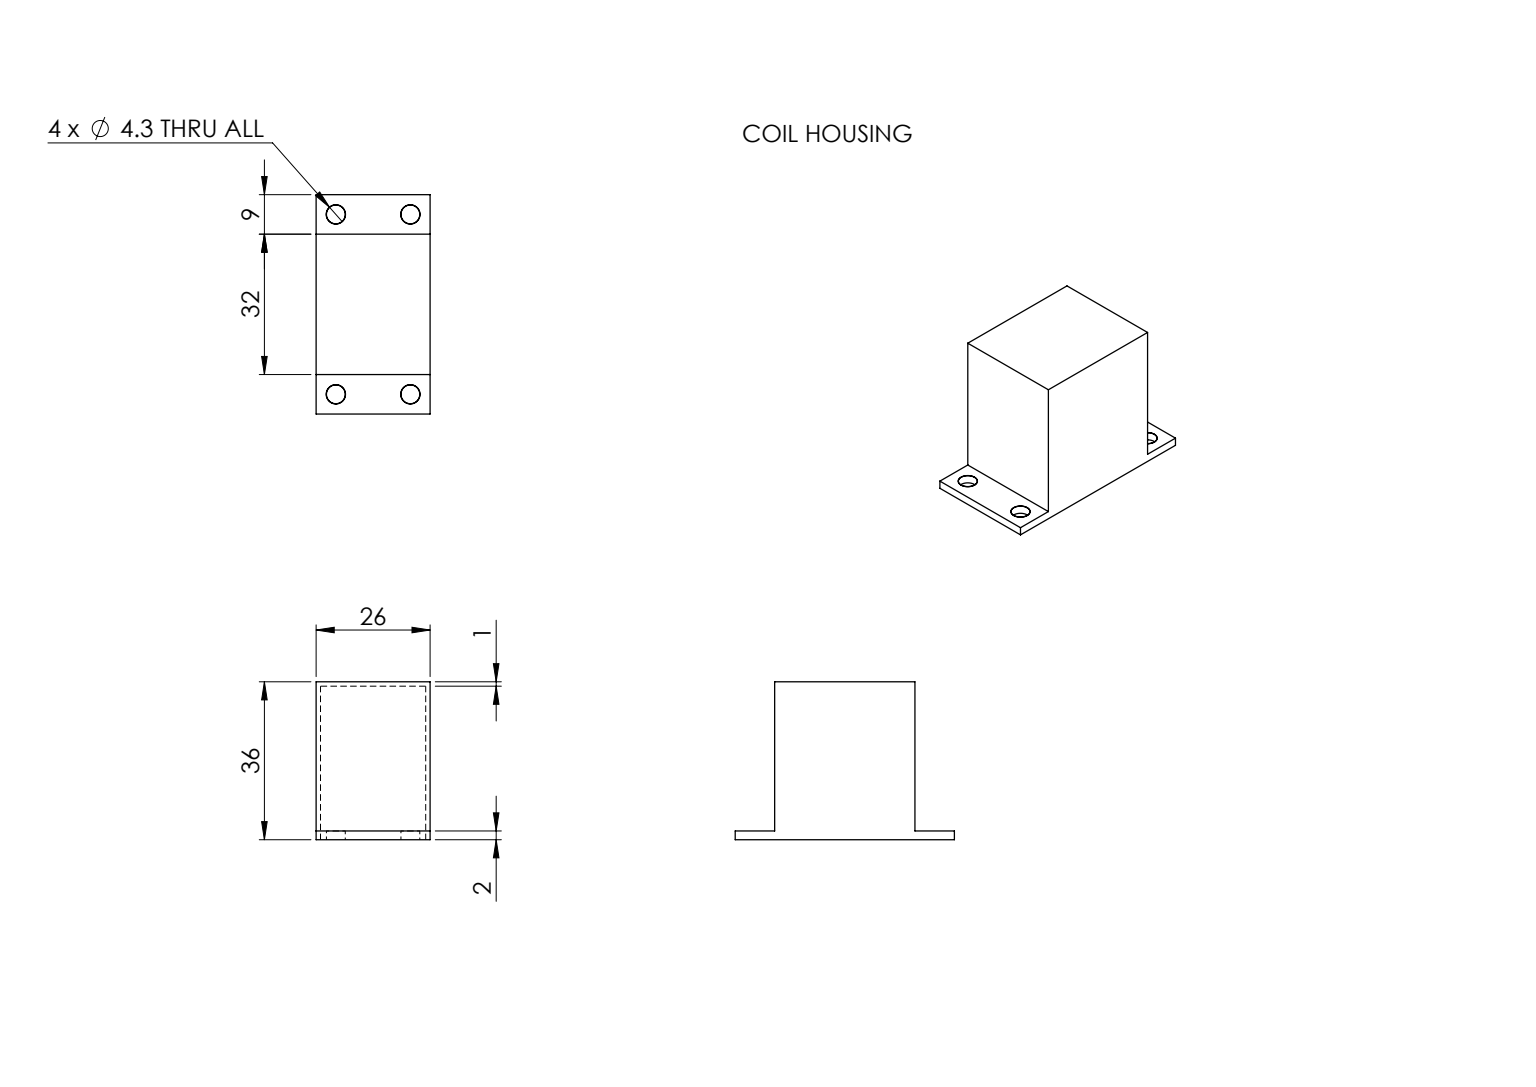
ISO-10303-21;
HEADER;
FILE_DESCRIPTION (('STEP AP214'),
    '1' );
FILE_NAME ('Coil Housing.step',
    '2026-10-25T16:39:07',
    ( '' ),
    ( '' ),
    'SwSTEP 2.0',
    'SolidWorks 2026',
    '' );
FILE_SCHEMA (( 'AUTOMOTIVE_DESIGN' ));
ENDSEC;

DATA;
#5=DIRECTION ( 'NONE',  ( -0.000000000000000000, 1.000000000000000000, -0.000000000000000000 ) ) ;
#11=LINE ( 'NONE', #8170, #4109 ) ;
#36=DIRECTION ( 'NONE',  ( 0.000000000000000000, 0.000000000000000000, 1.000000000000000000 ) ) ;
#41=CARTESIAN_POINT ( 'NONE',  ( -11.99999999999999822, 48.00000000000000000, 15.00000000000000000 ) ) ;
#55=ORIENTED_EDGE ( 'NONE', *, *, #17293, .T. ) ;
#160=VECTOR ( 'NONE', #10107, 1000.000000000000000 ) ;
#167=ORIENTED_EDGE ( 'NONE', *, *, #2613, .T. ) ;
#201=EDGE_CURVE ( 'NONE', #2949, #3217, #16754, .T. ) ;
#210=EDGE_CURVE ( 'NONE', #16170, #12849, #15356, .T. ) ;
#221=DIRECTION ( 'NONE',  ( -1.000000000000000000, 0.000000000000000000, 0.000000000000000000 ) ) ;
#243=CIRCLE ( 'NONE', #11190, 2.149999999999999023 ) ;
#258=DIRECTION ( 'NONE',  ( 0.000000000000000000, 0.000000000000000000, 1.000000000000000000 ) ) ;
#282=DIRECTION ( 'NONE',  ( 0.000000000000000000, 0.000000000000000000, -1.000000000000000000 ) ) ;
#297=VERTEX_POINT ( 'NONE', #12091 ) ;
#331=PLANE ( 'NONE',  #16743 ) ;
#386=FACE_OUTER_BOUND ( 'NONE', #16135, .T. ) ;
#409=ORIENTED_EDGE ( 'NONE', *, *, #7785, .F. ) ;
#452=DIRECTION ( 'NONE',  ( -0.000000000000000000, -0.000000000000000000, 1.000000000000000000 ) ) ;
#518=CARTESIAN_POINT ( 'NONE',  ( -8.500000000000007105, 14.80000000000000071, -20.49999999999999645 ) ) ;
#554=CARTESIAN_POINT ( 'NONE',  ( -8.500000000000007105, 15.00000000000000000, -20.49999999999999645 ) ) ;
#593=DIRECTION ( 'NONE',  ( 1.000000000000000000, 0.000000000000000000, 1.224646799147353207E-16 ) ) ;
#623=ORIENTED_EDGE ( 'NONE', *, *, #10806, .F. ) ;
#658=DIRECTION ( 'NONE',  ( 0.000000000000000000, 0.000000000000000000, 1.000000000000000000 ) ) ;
#706=DIRECTION ( 'NONE',  ( 0.000000000000000000, -0.000000000000000000, -1.000000000000000000 ) ) ;
#789=ADVANCED_FACE ( 'NONE', ( #9941 ), #12905, .F. ) ;
#800=ORIENTED_EDGE ( 'NONE', *, *, #7498, .F. ) ;
#842=EDGE_CURVE ( 'NONE', #9790, #6836, #12069, .T. ) ;
#872=ORIENTED_EDGE ( 'NONE', *, *, #16127, .F. ) ;
#958=DIRECTION ( 'NONE',  ( 0.000000000000000000, 0.000000000000000000, 1.000000000000000000 ) ) ;
#965=AXIS2_PLACEMENT_3D ( 'NONE', #17029, #8642, #1809 ) ;
#1016=TOROIDAL_SURFACE ( 'NONE', #15523, 2.200000000000000178, 0.2000000000000000111 ) ;
#1021=EDGE_LOOP ( 'NONE', ( #11107, #14324, #7812, #9618 ) ) ;
#1022=DIRECTION ( 'NONE',  ( -0.000000000000000000, 1.000000000000000000, -0.000000000000000000 ) ) ;
#1054=DIRECTION ( 'NONE',  ( -0.000000000000000000, 1.000000000000000000, -0.000000000000000000 ) ) ;
#1065=VECTOR ( 'NONE', #8366, 1000.000000000000000 ) ;
#1071=DIRECTION ( 'NONE',  ( -0.000000000000000000, 1.000000000000000000, -0.000000000000000000 ) ) ;
#1073=AXIS2_PLACEMENT_3D ( 'NONE', #1154, #15068, #6797 ) ;
#1078=CARTESIAN_POINT ( 'NONE',  ( 13.00000000000000178, 15.00000000000000178, -25.00000000000000355 ) ) ;
#1093=ORIENTED_EDGE ( 'NONE', *, *, #9929, .T. ) ;
#1099=FILL_AREA_STYLE ('',( #8400 ) ) ;
#1113=ADVANCED_FACE ( 'NONE', ( #1240 ), #4479, .T. ) ;
#1140=AXIS2_PLACEMENT_3D ( 'NONE', #6146, #11796, #10410 ) ;
#1154=CARTESIAN_POINT ( 'NONE',  ( -11.99999999999999822, 48.00000000000000000, -15.00000000000000000 ) ) ;
#1166=AXIS2_PLACEMENT_3D ( 'NONE', #8962, #12855, #8673 ) ;
#1183=DIRECTION ( 'NONE',  ( 0.000000000000000000, 0.000000000000000000, 1.000000000000000000 ) ) ;
#1194=SURFACE_STYLE_FILL_AREA ( #1099 ) ;
#1212=CARTESIAN_POINT ( 'NONE',  ( 8.500000000000001776, 13.00000000000000000, -22.64999999999999503 ) ) ;
#1216=FACE_OUTER_BOUND ( 'NONE', #16174, .T. ) ;
#1240=FACE_OUTER_BOUND ( 'NONE', #5632, .T. ) ;
#1252=ADVANCED_FACE ( 'NONE', ( #11227 ), #9922, .F. ) ;
#1254=DIRECTION ( 'NONE',  ( 1.000000000000000000, 0.000000000000000000, 0.000000000000000000 ) ) ;
#1264=CARTESIAN_POINT ( 'NONE',  ( -12.99999999999999822, 48.00000000000000000, -16.00000000000000000 ) ) ;
#1271=CARTESIAN_POINT ( 'NONE',  ( 8.500000000000001776, 14.99364916731036956, -20.49999999999999645 ) ) ;
#1277=EDGE_CURVE ( 'NONE', #11364, #9512, #18161, .T. ) ;
#1285=VERTEX_POINT ( 'NONE', #15594 ) ;
#1341=LINE ( 'NONE', #16656, #4429 ) ;
#1342=CYLINDRICAL_SURFACE ( 'NONE', #3202, 2.149999999999995470 ) ;
#1346=VERTEX_POINT ( 'NONE', #5580 ) ;
#1361=CARTESIAN_POINT ( 'NONE',  ( -8.500000000000010658, 14.99364916731036956, 18.34999999999999432 ) ) ;
#1362=AXIS2_PLACEMENT_3D ( 'NONE', #14070, #1651, #258 ) ;
#1388=ORIENTED_EDGE ( 'NONE', *, *, #14830, .T. ) ;
#1419=LINE ( 'NONE', #5668, #14928 ) ;
#1422=ORIENTED_EDGE ( 'NONE', *, *, #16477, .F. ) ;
#1456=CARTESIAN_POINT ( 'NONE',  ( -11.99999999999999822, 13.00000000000000178, -15.00000000000000000 ) ) ;
#1465=( LENGTH_UNIT ( ) NAMED_UNIT ( * ) SI_UNIT ( .MILLI., .METRE. ) );
#1466=DIRECTION ( 'NONE',  ( 1.000000000000000000, 0.000000000000000000, 0.000000000000000000 ) ) ;
#1468=ORIENTED_EDGE ( 'NONE', *, *, #10652, .T. ) ;
#1534=ORIENTED_EDGE ( 'NONE', *, *, #210, .T. ) ;
#1538=FACE_OUTER_BOUND ( 'NONE', #12873, .T. ) ;
#1551=FACE_OUTER_BOUND ( 'NONE', #4692, .T. ) ;
#1602=DIRECTION ( 'NONE',  ( -0.000000000000000000, 1.000000000000000000, -0.000000000000000000 ) ) ;
#1608=ADVANCED_FACE ( 'NONE', ( #1216 ), #3033, .T. ) ;
#1618=DIRECTION ( 'NONE',  ( 0.000000000000000000, 0.000000000000000000, 1.000000000000000000 ) ) ;
#1651=DIRECTION ( 'NONE',  ( -0.000000000000000000, 1.000000000000000000, -0.000000000000000000 ) ) ;
#1677=EDGE_CURVE ( 'NONE', #13721, #297, #14916, .T. ) ;
#1696=AXIS2_PLACEMENT_3D ( 'NONE', #10677, #16349, #958 ) ;
#1720=AXIS2_PLACEMENT_3D ( 'NONE', #7114, #5912, #15845 ) ;
#1733=VECTOR ( 'NONE', #3727, 1000.000000000000000 ) ;
#1761=VERTEX_POINT ( 'NONE', #17446 ) ;
#1765=VECTOR ( 'NONE', #16029, 1000.000000000000000 ) ;
#1789=DIRECTION ( 'NONE',  ( -0.000000000000000000, -1.000000000000000000, -0.000000000000000000 ) ) ;
#1809=DIRECTION ( 'NONE',  ( 0.000000000000000000, 0.000000000000000000, 1.000000000000000000 ) ) ;
#1819=DIRECTION ( 'NONE',  ( -0.000000000000000000, -1.000000000000000000, -0.000000000000000000 ) ) ;
#1884=EDGE_LOOP ( 'NONE', ( #14599, #5933, #16408, #14556 ) ) ;
#1885=STYLED_ITEM('',(#18389),#2427);
#1904=DIRECTION ( 'NONE',  ( -0.000000000000000000, -1.000000000000000000, -0.000000000000000000 ) ) ;
#1914=ORIENTED_EDGE ( 'NONE', *, *, #14897, .T. ) ;
#1942=FACE_OUTER_BOUND ( 'NONE', #17721, .T. ) ;
#1988=AXIS2_PLACEMENT_3D ( 'NONE', #15629, #5433, #11080 ) ;
#2022=DIRECTION ( 'NONE',  ( 0.000000000000000000, 0.000000000000000000, -1.000000000000000000 ) ) ;
#2058=DIRECTION ( 'NONE',  ( 1.000000000000000000, 0.000000000000000000, -0.000000000000000000 ) ) ;
#2063=CARTESIAN_POINT ( 'NONE',  ( 0.000000000000000000, 15.00000000000000178, 0.000000000000000000 ) ) ;
#2109=CARTESIAN_POINT ( 'NONE',  ( -12.99999999999999822, 48.00000000000000000, 16.00000000000000000 ) ) ;
#2150=ADVANCED_FACE ( 'NONE', ( #14013 ), #17441, .T. ) ;
#2189=CARTESIAN_POINT ( 'NONE',  ( -8.500000000000010658, 13.00000000000000000, 22.64999999999998437 ) ) ;
#2215=VERTEX_POINT ( 'NONE', #2810 ) ;
#2229=( LENGTH_UNIT ( ) NAMED_UNIT ( * ) SI_UNIT ( .MILLI., .METRE. ) );
#2242=EDGE_CURVE ( 'NONE', #6649, #8268, #1419, .T. ) ;
#2250=CARTESIAN_POINT ( 'NONE',  ( 8.499999999999992895, 14.80000000000000071, 20.49999999999999645 ) ) ;
#2266=DIRECTION ( 'NONE',  ( 0.000000000000000000, -1.000000000000000000, 0.000000000000000000 ) ) ;
#2310=CIRCLE ( 'NONE', #12648, 2.200000000000000622 ) ;
#2312=ADVANCED_FACE ( 'NONE', ( #7695 ), #13356, .F. ) ;
#2338=( LENGTH_UNIT ( ) NAMED_UNIT ( * ) SI_UNIT ( .MILLI., .METRE. ) );
#2378=CARTESIAN_POINT ( 'NONE',  ( 0.000000000000000000, 15.00000000000000178, 0.000000000000000000 ) ) ;
#2383=EDGE_CURVE ( 'NONE', #10239, #2662, #17878, .T. ) ;
#2403=VECTOR ( 'NONE', #17387, 1000.000000000000000 ) ;
#2408=( NAMED_UNIT ( * ) SI_UNIT ( $, .STERADIAN. ) SOLID_ANGLE_UNIT ( ) );
#2420=CARTESIAN_POINT ( 'NONE',  ( -8.500000000000010658, 13.00000000000000000, 20.49999999999998934 ) ) ;
#2421=DIRECTION ( 'NONE',  ( -0.000000000000000000, -1.000000000000000000, -0.000000000000000000 ) ) ;
#2425=FACE_OUTER_BOUND ( 'NONE', #4834, .T. ) ;
#2427=MANIFOLD_SOLID_BREP ( 'Cavity1', #15632 ) ;
#2469=CARTESIAN_POINT ( 'NONE',  ( -8.500000000000010658, 15.00000000000000178, 18.34999999999999432 ) ) ;
#2479=VECTOR ( 'NONE', #1789, 1000.000000000000000 ) ;
#2481=ORIENTED_EDGE ( 'NONE', *, *, #6992, .T. ) ;
#2500=DIRECTION ( 'NONE',  ( 0.000000000000000000, 0.000000000000000000, 1.000000000000000000 ) ) ;
#2503=LINE ( 'NONE', #16686, #9260 ) ;
#2535=CARTESIAN_POINT ( 'NONE',  ( 12.00000000000000178, 48.00000000000000000, 15.00000000000000000 ) ) ;
#2545=ORIENTED_EDGE ( 'NONE', *, *, #4076, .F. ) ;
#2552=DIRECTION ( 'NONE',  ( -0.000000000000000000, 1.000000000000000000, -0.000000000000000000 ) ) ;
#2553=CARTESIAN_POINT ( 'NONE',  ( 8.499999999999994671, 13.00000000000000000, 22.64999999999999503 ) ) ;
#2563=DIRECTION ( 'NONE',  ( 0.000000000000000000, -1.000000000000000000, 0.000000000000000000 ) ) ;
#2577=CARTESIAN_POINT ( 'NONE',  ( -8.500000000000010658, 14.80000000000000071, 20.49999999999998934 ) ) ;
#2597=ORIENTED_EDGE ( 'NONE', *, *, #842, .T. ) ;
#2598=CARTESIAN_POINT ( 'NONE',  ( -11.99999999999999822, 48.00000000000000000, 15.00000000000000000 ) ) ;
#2613=EDGE_CURVE ( 'NONE', #7280, #11197, #10033, .T. ) ;
#2652=EDGE_CURVE ( 'NONE', #13721, #9512, #7748, .T. ) ;
#2662=VERTEX_POINT ( 'NONE', #3290 ) ;
#2669=DIRECTION ( 'NONE',  ( 0.000000000000000000, 0.000000000000000000, 1.000000000000000000 ) ) ;
#2671=CARTESIAN_POINT ( 'NONE',  ( 8.499999999999994671, 14.99364916731036956, 22.64999999999999147 ) ) ;
#2679=SHAPE_REPRESENTATION_RELATIONSHIP ( 'NONE' , 'NONE' ,  #10877, #16698 ) ;
#2688=EDGE_CURVE ( 'NONE', #2662, #16507, #13972, .T. ) ;
#2698=CARTESIAN_POINT ( 'NONE',  ( 0.000000000000000000, 48.00000000000000000, 0.000000000000000000 ) ) ;
#2699=ORIENTED_EDGE ( 'NONE', *, *, #6147, .F. ) ;
#2721=CARTESIAN_POINT ( 'NONE',  ( -8.500000000000005329, 15.00000000000000178, -20.49999999999999645 ) ) ;
#2738=LINE ( 'NONE', #2469, #17193 ) ;
#2772=CARTESIAN_POINT ( 'NONE',  ( -13.00000000000000178, 15.00000000000000178, -25.00000000000000355 ) ) ;
#2775=ORIENTED_EDGE ( 'NONE', *, *, #17964, .T. ) ;
#2786=DIRECTION ( 'NONE',  ( 0.000000000000000000, -0.000000000000000000, -1.000000000000000000 ) ) ;
#2810=CARTESIAN_POINT ( 'NONE',  ( -13.00000000000000178, 15.00000000000000178, 25.00000000000000355 ) ) ;
#2812=DIRECTION ( 'NONE',  ( 0.000000000000000000, 0.000000000000000000, 1.000000000000000000 ) ) ;
#2844=VERTEX_POINT ( 'NONE', #7317 ) ;
#2889=DIRECTION ( 'NONE',  ( -0.000000000000000000, 1.000000000000000000, -0.000000000000000000 ) ) ;
#2909=CARTESIAN_POINT ( 'NONE',  ( 8.500000000000000000, 15.00000000000000000, -22.69999999999999929 ) ) ;
#2949=VERTEX_POINT ( 'NONE', #14676 ) ;
#2954=CARTESIAN_POINT ( 'NONE',  ( -11.99999999999999822, 48.00000000000000000, 15.00000000000000000 ) ) ;
#3012=CIRCLE ( 'NONE', #17864, 2.149999999999995470 ) ;
#3033=TOROIDAL_SURFACE ( 'NONE', #12497, 2.200000000000000178, 0.2000000000000000111 ) ;
#3038=ORIENTED_EDGE ( 'NONE', *, *, #16535, .T. ) ;
#3041=EDGE_CURVE ( 'NONE', #9856, #16492, #12322, .T. ) ;
#3042=ORIENTED_EDGE ( 'NONE', *, *, #1277, .T. ) ;
#3084=DIRECTION ( 'NONE',  ( 0.000000000000000000, 0.000000000000000000, 1.000000000000000000 ) ) ;
#3098=EDGE_LOOP ( 'NONE', ( #17464, #3426, #5820, #17938 ) ) ;
#3121=ORIENTED_EDGE ( 'NONE', *, *, #7037, .T. ) ;
#3170=ORIENTED_EDGE ( 'NONE', *, *, #10062, .T. ) ;
#3172=LINE ( 'NONE', #1264, #2479 ) ;
#3183=AXIS2_PLACEMENT_3D ( 'NONE', #2698, #11198, #2786 ) ;
#3184=DIRECTION ( 'NONE',  ( 0.000000000000000000, -1.000000000000000000, 0.000000000000000000 ) ) ;
#3185=VERTEX_POINT ( 'NONE', #10264 ) ;
#3190=FACE_OUTER_BOUND ( 'NONE', #10306, .T. ) ;
#3193=DIRECTION ( 'NONE',  ( 0.000000000000000000, -1.000000000000000000, 0.000000000000000000 ) ) ;
#3202=AXIS2_PLACEMENT_3D ( 'NONE', #8544, #15351, #17105 ) ;
#3209=DIRECTION ( 'NONE',  ( 0.000000000000000000, 0.000000000000000000, 1.000000000000000000 ) ) ;
#3217=VERTEX_POINT ( 'NONE', #6005 ) ;
#3239=ORIENTED_EDGE ( 'NONE', *, *, #2688, .F. ) ;
#3250=ORIENTED_EDGE ( 'NONE', *, *, #5910, .T. ) ;
#3290=CARTESIAN_POINT ( 'NONE',  ( 8.500000000000001776, 15.00000000000000000, -18.29999999999999716 ) ) ;
#3296=DIRECTION ( 'NONE',  ( 1.000000000000000000, 0.000000000000000000, -0.000000000000000000 ) ) ;
#3334=ORIENTED_EDGE ( 'NONE', *, *, #14608, .T. ) ;
#3340=ORIENTED_EDGE ( 'NONE', *, *, #12040, .T. ) ;
#3360=MECHANICAL_DESIGN_GEOMETRIC_PRESENTATION_REPRESENTATION('',(#1885),#7184);
#3381=ORIENTED_EDGE ( 'NONE', *, *, #14211, .F. ) ;
#3387=VECTOR ( 'NONE', #2552, 1000.000000000000000 ) ;
#3421=VERTEX_POINT ( 'NONE', #4810 ) ;
#3426=ORIENTED_EDGE ( 'NONE', *, *, #11240, .T. ) ;
#3440=EDGE_CURVE ( 'NONE', #5643, #9512, #12120, .T. ) ;
#3454=EDGE_CURVE ( 'NONE', #15329, #1285, #6590, .T. ) ;
#3534=DIRECTION ( 'NONE',  ( 0.000000000000000000, -0.000000000000000000, -1.000000000000000000 ) ) ;
#3598=ORIENTED_EDGE ( 'NONE', *, *, #4237, .T. ) ;
#3601=EDGE_CURVE ( 'NONE', #9347, #10311, #5169, .T. ) ;
#3625=DIRECTION ( 'NONE',  ( -0.000000000000000000, 1.000000000000000000, -0.000000000000000000 ) ) ;
#3635=AXIS2_PLACEMENT_3D ( 'NONE', #13994, #9900, #5554 ) ;
#3665=FACE_BOUND ( 'NONE', #3976, .T. ) ;
#3676=DIRECTION ( 'NONE',  ( 1.000000000000000000, 0.000000000000000000, 1.224646799147353207E-16 ) ) ;
#3682=CARTESIAN_POINT ( 'NONE',  ( -8.500000000000005329, 15.00000000000000178, -20.49999999999999645 ) ) ;
#3684=DIRECTION ( 'NONE',  ( 0.000000000000000000, 0.000000000000000000, -1.000000000000000000 ) ) ;
#3727=DIRECTION ( 'NONE',  ( -0.000000000000000000, 1.000000000000000000, -0.000000000000000000 ) ) ;
#3740=PLANE ( 'NONE',  #1073 ) ;
#3765=CYLINDRICAL_SURFACE ( 'NONE', #4714, 2.149999999999995470 ) ;
#3770=ORIENTED_EDGE ( 'NONE', *, *, #3041, .T. ) ;
#3778=( NAMED_UNIT ( * ) PLANE_ANGLE_UNIT ( ) SI_UNIT ( $, .RADIAN. ) );
#3790=LINE ( 'NONE', #15115, #18269 ) ;
#3818=ORIENTED_EDGE ( 'NONE', *, *, #12155, .T. ) ;
#3837=AXIS2_PLACEMENT_3D ( 'NONE', #11609, #8636, #36 ) ;
#3838=CARTESIAN_POINT ( 'NONE',  ( -13.00000000000000178, 49.00000000000000000, -16.00000000000000000 ) ) ;
#3883=VECTOR ( 'NONE', #15541, 1000.000000000000000 ) ;
#3904=ORIENTED_EDGE ( 'NONE', *, *, #7785, .T. ) ;
#3911=CYLINDRICAL_SURFACE ( 'NONE', #16250, 2.149999999999995470 ) ;
#3926=CARTESIAN_POINT ( 'NONE',  ( 8.500000000000001776, 14.99364916731036956, -22.64999999999999147 ) ) ;
#3933=FACE_OUTER_BOUND ( 'NONE', #1021, .T. ) ;
#3944=AXIS2_PLACEMENT_3D ( 'NONE', #17372, #10383, #9272 ) ;
#3976=EDGE_LOOP ( 'NONE', ( #17391, #409 ) ) ;
#3994=ORIENTED_EDGE ( 'NONE', *, *, #12650, .F. ) ;
#4010=DIRECTION ( 'NONE',  ( 0.000000000000000000, 0.000000000000000000, 1.000000000000000000 ) ) ;
#4022=CARTESIAN_POINT ( 'NONE',  ( -13.00000000000000178, 15.00000000000000178, -25.00000000000000355 ) ) ;
#4035=VECTOR ( 'NONE', #15160, 1000.000000000000000 ) ;
#4038=CARTESIAN_POINT ( 'NONE',  ( 8.499999999999992895, 14.80000000000000071, 22.69999999999999929 ) ) ;
#4062=VECTOR ( 'NONE', #16950, 1000.000000000000000 ) ;
#4065=PLANE ( 'NONE',  #3183 ) ;
#4069=( NAMED_UNIT ( * ) PLANE_ANGLE_UNIT ( ) SI_UNIT ( $, .RADIAN. ) );
#4071=ORIENTED_EDGE ( 'NONE', *, *, #6036, .F. ) ;
#4076=EDGE_CURVE ( 'NONE', #13129, #6514, #11073, .T. ) ;
#4104=LINE ( 'NONE', #12809, #1065 ) ;
#4109=VECTOR ( 'NONE', #6956, 1000.000000000000000 ) ;
#4135=CARTESIAN_POINT ( 'NONE',  ( 13.00000000000000178, 15.00000000000000178, 16.00000000000000000 ) ) ;
#4225=CARTESIAN_POINT ( 'NONE',  ( 13.00000000000000178, 49.00000000000000000, 16.00000000000000000 ) ) ;
#4237=EDGE_CURVE ( 'NONE', #4992, #6649, #3172, .T. ) ;
#4266=ORIENTED_EDGE ( 'NONE', *, *, #2242, .F. ) ;
#4267=DIRECTION ( 'NONE',  ( 0.000000000000000000, 0.000000000000000000, 1.000000000000000000 ) ) ;
#4280=DIRECTION ( 'NONE',  ( 0.000000000000000000, 0.000000000000000000, 1.000000000000000000 ) ) ;
#4286=LINE ( 'NONE', #9931, #160 ) ;
#4295=CARTESIAN_POINT ( 'NONE',  ( -13.00000000000000178, 49.00000000000000000, 16.00000000000000000 ) ) ;
#4319=SURFACE_STYLE_USAGE ( .BOTH. , #7095 ) ;
#4337=ORIENTED_EDGE ( 'NONE', *, *, #16762, .F. ) ;
#4365=AXIS2_PLACEMENT_3D ( 'NONE', #10794, #1071, #8008 ) ;
#4372=VECTOR ( 'NONE', #6715, 1000.000000000000000 ) ;
#4380=DIRECTION ( 'NONE',  ( -0.000000000000000000, -1.000000000000000000, -0.000000000000000000 ) ) ;
#4385=EDGE_LOOP ( 'NONE', ( #2545, #13867, #3250, #11309 ) ) ;
#4391=TOROIDAL_SURFACE ( 'NONE', #12673, 2.200000000000000178, 0.2000000000000000111 ) ;
#4429=VECTOR ( 'NONE', #12360, 1000.000000000000000 ) ;
#4479=TOROIDAL_SURFACE ( 'NONE', #17239, 2.200000000000000178, 0.2000000000000000111 ) ;
#4494=FACE_OUTER_BOUND ( 'NONE', #13704, .T. ) ;
#4520=LINE ( 'NONE', #11457, #17177 ) ;
#4565=LINE ( 'NONE', #12731, #2403 ) ;
#4633=CARTESIAN_POINT ( 'NONE',  ( -8.500000000000005329, 14.99364916731036956, -18.35000000000000142 ) ) ;
#4651=EDGE_CURVE ( 'NONE', #6401, #11263, #2503, .T. ) ;
#4684=VECTOR ( 'NONE', #282, 1000.000000000000000 ) ;
#4692=EDGE_LOOP ( 'NONE', ( #13063, #15901, #167, #9863 ) ) ;
#4710=VERTEX_POINT ( 'NONE', #2772 ) ;
#4714=AXIS2_PLACEMENT_3D ( 'NONE', #13224, #11834, #4795 ) ;
#4755=ORIENTED_EDGE ( 'NONE', *, *, #3440, .T. ) ;
#4758=APPLICATION_CONTEXT ( 'automotive_design' ) ;
#4759=ORIENTED_EDGE ( 'NONE', *, *, #2383, .F. ) ;
#4770=DIRECTION ( 'NONE',  ( -0.000000000000000000, 1.000000000000000000, -0.000000000000000000 ) ) ;
#4778=ORIENTED_EDGE ( 'NONE', *, *, #5020, .F. ) ;
#4795=DIRECTION ( 'NONE',  ( 0.000000000000000000, 0.000000000000000000, 1.000000000000000000 ) ) ;
#4801=ADVANCED_FACE ( 'NONE', ( #1551 ), #9965, .T. ) ;
#4807=DIRECTION ( 'NONE',  ( 0.000000000000000000, 0.000000000000000000, 1.000000000000000000 ) ) ;
#4810=CARTESIAN_POINT ( 'NONE',  ( -13.00000000000000178, 15.00000000000000178, 16.00000000000000000 ) ) ;
#4817=ORIENTED_EDGE ( 'NONE', *, *, #1277, .F. ) ;
#4823=DIRECTION ( 'NONE',  ( -0.000000000000000000, 1.000000000000000000, -0.000000000000000000 ) ) ;
#4831=CARTESIAN_POINT ( 'NONE',  ( 8.500000000000001776, 15.00000000000000000, -20.49999999999999645 ) ) ;
#4834=EDGE_LOOP ( 'NONE', ( #14359, #2699, #623, #14473 ) ) ;
#4845=AXIS2_PLACEMENT_3D ( 'NONE', #17879, #6540, #5148 ) ;
#4884=EDGE_CURVE ( 'NONE', #15656, #6744, #12847, .T. ) ;
#4891=ORIENTED_EDGE ( 'NONE', *, *, #11809, .T. ) ;
#4895=VERTEX_POINT ( 'NONE', #5803 ) ;
#4918=DIRECTION ( 'NONE',  ( -0.000000000000000000, 1.000000000000000000, -0.000000000000000000 ) ) ;
#4975=CARTESIAN_POINT ( 'NONE',  ( 8.500000000000001776, 15.00000000000000178, -20.49999999999999645 ) ) ;
#4992=VERTEX_POINT ( 'NONE', #12006 ) ;
#5020=EDGE_CURVE ( 'NONE', #10239, #6514, #12232, .T. ) ;
#5148=DIRECTION ( 'NONE',  ( 0.000000000000000000, 0.000000000000000000, 1.000000000000000000 ) ) ;
#5169=LINE ( 'NONE', #18175, #12206 ) ;
#5173=ORIENTED_EDGE ( 'NONE', *, *, #6036, .T. ) ;
#5221=LINE ( 'NONE', #9481, #3387 ) ;
#5240=ADVANCED_FACE ( 'NONE', ( #14995 ), #13769, .F. ) ;
#5260=CIRCLE ( 'NONE', #9695, 2.149999999999999023 ) ;
#5293=VERTEX_POINT ( 'NONE', #11158 ) ;
#5318=FACE_OUTER_BOUND ( 'NONE', #17771, .T. ) ;
#5319=CIRCLE ( 'NONE', #11217, 2.149999999999999023 ) ;
#5371=CARTESIAN_POINT ( 'NONE',  ( -11.99999999999999822, 48.00000000000000000, 15.00000000000000000 ) ) ;
#5387=VECTOR ( 'NONE', #15492, 1000.000000000000000 ) ;
#5433=DIRECTION ( 'NONE',  ( -0.000000000000000000, 1.000000000000000000, -0.000000000000000000 ) ) ;
#5487=ORIENTED_EDGE ( 'NONE', *, *, #9824, .F. ) ;
#5492=ORIENTED_EDGE ( 'NONE', *, *, #13638, .T. ) ;
#5526=EDGE_LOOP ( 'NONE', ( #13577, #4759 ) ) ;
#5551=ORIENTED_EDGE ( 'NONE', *, *, #210, .F. ) ;
#5554=DIRECTION ( 'NONE',  ( 0.000000000000000000, 0.000000000000000000, 1.000000000000000000 ) ) ;
#5562=VECTOR ( 'NONE', #4380, 1000.000000000000000 ) ;
#5580=CARTESIAN_POINT ( 'NONE',  ( 8.499999999999994671, 14.99364916731036956, 18.35000000000000142 ) ) ;
#5599=PRODUCT_DEFINITION ( 'UNKNOWN', '', #9538, #12661 ) ;
#5627=AXIS2_PLACEMENT_3D ( 'NONE', #8566, #13021, #13116 ) ;
#5632=EDGE_LOOP ( 'NONE', ( #5492, #13247, #12663, #3239 ) ) ;
#5643=VERTEX_POINT ( 'NONE', #2189 ) ;
#5668=CARTESIAN_POINT ( 'NONE',  ( -13.00000000000000178, 15.00000000000000178, -16.00000000000000000 ) ) ;
#5679=STYLED_ITEM ( 'NONE', ( #9793 ), #16698 ) ;
#5735=ORIENTED_EDGE ( 'NONE', *, *, #6017, .F. ) ;
#5756=LINE ( 'NONE', #17348, #8903 ) ;
#5759=ORIENTED_EDGE ( 'NONE', *, *, #2652, .T. ) ;
#5803=CARTESIAN_POINT ( 'NONE',  ( 8.499999999999994671, 13.00000000000000000, 18.34999999999999787 ) ) ;
#5820=ORIENTED_EDGE ( 'NONE', *, *, #7161, .F. ) ;
#5902=ADVANCED_FACE ( 'NONE', ( #5318 ), #1016, .T. ) ;
#5910=EDGE_CURVE ( 'NONE', #1761, #16507, #5221, .T. ) ;
#5912=DIRECTION ( 'NONE',  ( 1.000000000000000000, 0.000000000000000000, 1.224646799147353207E-16 ) ) ;
#5933=ORIENTED_EDGE ( 'NONE', *, *, #4076, .T. ) ;
#5936=DIRECTION ( 'NONE',  ( 0.000000000000000000, 0.000000000000000000, -1.000000000000000000 ) ) ;
#5968=CARTESIAN_POINT ( 'NONE',  ( 13.00000000000000178, 15.00000000000000178, -16.00000000000000000 ) ) ;
#5971=CARTESIAN_POINT ( 'NONE',  ( -11.99999999999999822, 48.00000000000000000, -15.00000000000000000 ) ) ;
#6005=CARTESIAN_POINT ( 'NONE',  ( 13.00000000000000178, 13.00000000000000178, -25.00000000000000355 ) ) ;
#6010=EDGE_CURVE ( 'NONE', #14506, #15334, #14986, .T. ) ;
#6017=EDGE_CURVE ( 'NONE', #6744, #3421, #4104, .T. ) ;
#6036=EDGE_CURVE ( 'NONE', #10707, #2844, #4286, .T. ) ;
#6085=VECTOR ( 'NONE', #14166, 1000.000000000000000 ) ;
#6097=ORIENTED_EDGE ( 'NONE', *, *, #14830, .F. ) ;
#6103=CIRCLE ( 'NONE', #16486, 2.200000000000000622 ) ;
#6107=EDGE_CURVE ( 'NONE', #3217, #9347, #15521, .T. ) ;
#6113=DIRECTION ( 'NONE',  ( 0.000000000000000000, -0.000000000000000000, 1.000000000000000000 ) ) ;
#6146=CARTESIAN_POINT ( 'NONE',  ( 0.000000000000000000, 13.00000000000000178, 0.000000000000000000 ) ) ;
#6147=EDGE_CURVE ( 'NONE', #10707, #9790, #7523, .T. ) ;
#6273=VERTEX_POINT ( 'NONE', #16821 ) ;
#6290=DIRECTION ( 'NONE',  ( 0.000000000000000000, 0.000000000000000000, 1.000000000000000000 ) ) ;
#6310=FACE_BOUND ( 'NONE', #8681, .T. ) ;
#6331=AXIS2_PLACEMENT_3D ( 'NONE', #10056, #1466, #7190 ) ;
#6340=ORIENTED_EDGE ( 'NONE', *, *, #12494, .F. ) ;
#6395=CARTESIAN_POINT ( 'NONE',  ( -11.99999999999999822, 48.00000000000000000, -15.00000000000000000 ) ) ;
#6401=VERTEX_POINT ( 'NONE', #2553 ) ;
#6418=CARTESIAN_POINT ( 'NONE',  ( -8.500000000000010658, 14.80000000000000071, 18.29999999999999005 ) ) ;
#6422=ORIENTED_EDGE ( 'NONE', *, *, #13298, .F. ) ;
#6428=DIRECTION ( 'NONE',  ( 1.000000000000000000, 0.000000000000000000, 0.000000000000000000 ) ) ;
#6473=ORIENTED_EDGE ( 'NONE', *, *, #10561, .F. ) ;
#6479=DIRECTION ( 'NONE',  ( 0.000000000000000000, -1.000000000000000000, 0.000000000000000000 ) ) ;
#6486=PRODUCT ( 'Coil Housing', 'Coil Housing', '', ( #17700 ) ) ;
#6488=AXIS2_PLACEMENT_3D ( 'NONE', #3682, #17886, #13324 ) ;
#6514=VERTEX_POINT ( 'NONE', #3926 ) ;
#6530=DIRECTION ( 'NONE',  ( 0.000000000000000000, 0.000000000000000000, 1.000000000000000000 ) ) ;
#6540=DIRECTION ( 'NONE',  ( -0.000000000000000000, 1.000000000000000000, -0.000000000000000000 ) ) ;
#6575=AXIS2_PLACEMENT_3D ( 'NONE', #11492, #9837, #12712 ) ;
#6589=ADVANCED_FACE ( 'NONE', ( #9757 ), #3740, .T. ) ;
#6590=CIRCLE ( 'NONE', #11603, 2.200000000000000622 ) ;
#6608=DIRECTION ( 'NONE',  ( 0.000000000000000000, 0.000000000000000000, 1.000000000000000000 ) ) ;
#6619=DIRECTION ( 'NONE',  ( -0.000000000000000000, 1.000000000000000000, -0.000000000000000000 ) ) ;
#6634=DIRECTION ( 'NONE',  ( -0.000000000000000000, 1.000000000000000000, -0.000000000000000000 ) ) ;
#6649=VERTEX_POINT ( 'NONE', #8447 ) ;
#6658=ORIENTED_EDGE ( 'NONE', *, *, #13615, .T. ) ;
#6708=DIRECTION ( 'NONE',  ( 0.000000000000000000, -1.000000000000000000, 0.000000000000000000 ) ) ;
#6715=DIRECTION ( 'NONE',  ( -0.000000000000000000, -1.000000000000000000, -0.000000000000000000 ) ) ;
#6744=VERTEX_POINT ( 'NONE', #17196 ) ;
#6752=DIRECTION ( 'NONE',  ( 0.000000000000000000, 0.000000000000000000, -1.000000000000000000 ) ) ;
#6776=DIRECTION ( 'NONE',  ( 1.000000000000000000, 0.000000000000000000, 0.000000000000000000 ) ) ;
#6797=DIRECTION ( 'NONE',  ( 1.000000000000000000, 0.000000000000000000, 0.000000000000000000 ) ) ;
#6820=DIRECTION ( 'NONE',  ( -0.000000000000000000, 1.000000000000000000, -0.000000000000000000 ) ) ;
#6836=VERTEX_POINT ( 'NONE', #9910 ) ;
#6849=ORIENTED_EDGE ( 'NONE', *, *, #9077, .T. ) ;
#6868=FACE_OUTER_BOUND ( 'NONE', #7471, .T. ) ;
#6933=ORIENTED_EDGE ( 'NONE', *, *, #13615, .F. ) ;
#6934=EDGE_CURVE ( 'NONE', #13129, #1761, #243, .T. ) ;
#6935=DIRECTION ( 'NONE',  ( 0.000000000000000000, 0.000000000000000000, 1.000000000000000000 ) ) ;
#6956=DIRECTION ( 'NONE',  ( 0.000000000000000000, 0.000000000000000000, -1.000000000000000000 ) ) ;
#6963=CARTESIAN_POINT ( 'NONE',  ( 8.499999999999992895, 14.80000000000000071, 20.49999999999999645 ) ) ;
#6972=DIRECTION ( 'NONE',  ( -0.000000000000000000, 1.000000000000000000, -0.000000000000000000 ) ) ;
#6990=FACE_OUTER_BOUND ( 'NONE', #13889, .T. ) ;
#6992=EDGE_CURVE ( 'NONE', #2844, #6836, #7219, .T. ) ;
#7013=AXIS2_PLACEMENT_3D ( 'NONE', #4038, #9688, #13962 ) ;
#7037=EDGE_CURVE ( 'NONE', #4895, #6401, #7060, .T. ) ;
#7060=CIRCLE ( 'NONE', #9726, 2.149999999999999023 ) ;
#7095=SURFACE_SIDE_STYLE ('',( #1194 ) ) ;
#7104=ORIENTED_EDGE ( 'NONE', *, *, #17293, .F. ) ;
#7110=PLANE ( 'NONE',  #17783 ) ;
#7114=CARTESIAN_POINT ( 'NONE',  ( -8.500000000000007105, 14.80000000000000071, -22.69999999999999929 ) ) ;
#7156=EDGE_CURVE ( 'NONE', #5293, #17312, #7686, .T. ) ;
#7161=EDGE_CURVE ( 'NONE', #11263, #1346, #10032, .T. ) ;
#7180=VECTOR ( 'NONE', #16055, 1000.000000000000000 ) ;
#7184=( GEOMETRIC_REPRESENTATION_CONTEXT ( 3 ) GLOBAL_UNCERTAINTY_ASSIGNED_CONTEXT ( ( #18263 ) ) GLOBAL_UNIT_ASSIGNED_CONTEXT ( ( #2338, #4069, #7874 ) ) REPRESENTATION_CONTEXT ( 'NONE', 'WORKASPACE' ) );
#7190=DIRECTION ( 'NONE',  ( 0.000000000000000000, 0.000000000000000000, -1.000000000000000000 ) ) ;
#7215=ORIENTED_EDGE ( 'NONE', *, *, #6010, .T. ) ;
#7219=LINE ( 'NONE', #11298, #4684 ) ;
#7280=VERTEX_POINT ( 'NONE', #6395 ) ;
#7317=CARTESIAN_POINT ( 'NONE',  ( 12.00000000000000178, 13.00000000000000178, 15.00000000000000000 ) ) ;
#7343=FACE_BOUND ( 'NONE', #16900, .T. ) ;
#7353=ORIENTED_EDGE ( 'NONE', *, *, #9800, .F. ) ;
#7381=CARTESIAN_POINT ( 'NONE',  ( -13.00000000000000178, 49.00000000000000000, 16.00000000000000000 ) ) ;
#7393=EDGE_LOOP ( 'NONE', ( #5735, #7617, #15124, #2775 ) ) ;
#7437=EDGE_CURVE ( 'NONE', #1761, #13129, #5319, .T. ) ;
#7458=DIRECTION ( 'NONE',  ( -0.000000000000000000, 1.000000000000000000, -0.000000000000000000 ) ) ;
#7471=EDGE_LOOP ( 'NONE', ( #3381, #16000, #10596, #6340 ) ) ;
#7474=ORIENTED_EDGE ( 'NONE', *, *, #8857, .T. ) ;
#7498=EDGE_CURVE ( 'NONE', #11197, #17312, #8323, .T. ) ;
#7502=PLANE ( 'NONE',  #11652 ) ;
#7509=FACE_BOUND ( 'NONE', #5526, .T. ) ;
#7523=LINE ( 'NONE', #16163, #17366 ) ;
#7535=PLANE ( 'NONE',  #1140 ) ;
#7549=CARTESIAN_POINT ( 'NONE',  ( 8.499999999999994671, 13.00000000000000000, 20.49999999999999645 ) ) ;
#7577=CARTESIAN_POINT ( 'NONE',  ( -8.500000000000010658, 15.00000000000000000, 22.69999999999999218 ) ) ;
#7617=ORIENTED_EDGE ( 'NONE', *, *, #4884, .F. ) ;
#7675=AXIS2_PLACEMENT_3D ( 'NONE', #12019, #3684, #11933 ) ;
#7678=VECTOR ( 'NONE', #8232, 1000.000000000000000 ) ;
#7686=LINE ( 'NONE', #10275, #16278 ) ;
#7688=LINE ( 'NONE', #17650, #7180 ) ;
#7695=FACE_OUTER_BOUND ( 'NONE', #13374, .T. ) ;
#7728=DIRECTION ( 'NONE',  ( 0.000000000000000000, 0.000000000000000000, 1.000000000000000000 ) ) ;
#7748=CIRCLE ( 'NONE', #17250, 0.1999999999999987899 ) ;
#7785=EDGE_CURVE ( 'NONE', #297, #13721, #8959, .T. ) ;
#7808=ORIENTED_EDGE ( 'NONE', *, *, #12676, .F. ) ;
#7812=ORIENTED_EDGE ( 'NONE', *, *, #12676, .T. ) ;
#7854=EDGE_LOOP ( 'NONE', ( #15580, #11538, #8532, #1093 ) ) ;
#7874=( NAMED_UNIT ( * ) SI_UNIT ( $, .STERADIAN. ) SOLID_ANGLE_UNIT ( ) );
#7875=DIRECTION ( 'NONE',  ( 0.000000000000000000, 0.000000000000000000, 1.000000000000000000 ) ) ;
#7917=LINE ( 'NONE', #2109, #11871 ) ;
#7956=EDGE_LOOP ( 'NONE', ( #14367, #4071, #8081, #2597 ) ) ;
#7990=CARTESIAN_POINT ( 'NONE',  ( 8.500000000000001776, 14.80000000000000071, -20.49999999999999645 ) ) ;
#8000=CARTESIAN_POINT ( 'NONE',  ( -8.500000000000007105, 14.80000000000000071, -20.49999999999999645 ) ) ;
#8008=DIRECTION ( 'NONE',  ( 0.000000000000000000, 0.000000000000000000, 1.000000000000000000 ) ) ;
#8052=AXIS2_PLACEMENT_3D ( 'NONE', #8616, #5936, #17090 ) ;
#8081=ORIENTED_EDGE ( 'NONE', *, *, #6147, .T. ) ;
#8122=CARTESIAN_POINT ( 'NONE',  ( -11.99999999999999822, 48.00000000000000000, 15.00000000000000000 ) ) ;
#8128=EDGE_LOOP ( 'NONE', ( #17895, #3121 ) ) ;
#8139=VERTEX_POINT ( 'NONE', #11345 ) ;
#8165=CIRCLE ( 'NONE', #1362, 2.200000000000000622 ) ;
#8168=EDGE_CURVE ( 'NONE', #4710, #6649, #9684, .T. ) ;
#8170=CARTESIAN_POINT ( 'NONE',  ( 13.00000000000000178, 13.00000000000000178, 0.000000000000000000 ) ) ;
#8190=EDGE_CURVE ( 'NONE', #6514, #16507, #3012, .T. ) ;
#8230=ORIENTED_EDGE ( 'NONE', *, *, #12650, .T. ) ;
#8232=DIRECTION ( 'NONE',  ( -0.000000000000000000, -1.000000000000000000, -0.000000000000000000 ) ) ;
#8233=ADVANCED_FACE ( 'NONE', ( #1538 ), #331, .F. ) ;
#8268=VERTEX_POINT ( 'NONE', #5968 ) ;
#8295=EDGE_CURVE ( 'NONE', #8139, #8268, #14418, .T. ) ;
#8323=LINE ( 'NONE', #2598, #7678 ) ;
#8329=CARTESIAN_POINT ( 'NONE',  ( 8.499999999999992895, 15.00000000000000000, 20.49999999999999645 ) ) ;
#8335=COLOUR_RGB ( '',0.8941176470588234615, 0.8941176470588234615, 0.8941176470588234615 ) ;
#8366=DIRECTION ( 'NONE',  ( -1.000000000000000000, -0.000000000000000000, -0.000000000000000000 ) ) ;
#8386=CARTESIAN_POINT ( 'NONE',  ( 8.499999999999992895, 15.00000000000000000, 20.49999999999999645 ) ) ;
#8400=FILL_AREA_STYLE_COLOUR ( '', #8335 ) ;
#8435=DIRECTION ( 'NONE',  ( -0.000000000000000000, 1.000000000000000000, -0.000000000000000000 ) ) ;
#8447=CARTESIAN_POINT ( 'NONE',  ( -12.99999999999999822, 15.00000000000000000, -16.00000000000000000 ) ) ;
#8492=LINE ( 'NONE', #7381, #6085 ) ;
#8532=ORIENTED_EDGE ( 'NONE', *, *, #16511, .T. ) ;
#8544=CARTESIAN_POINT ( 'NONE',  ( -8.500000000000010658, 15.00000000000000178, 20.49999999999998934 ) ) ;
#8554=CARTESIAN_POINT ( 'NONE',  ( -13.00000000000000178, 13.00000000000000178, -25.00000000000000355 ) ) ;
#8562=DIRECTION ( 'NONE',  ( 0.000000000000000000, 0.000000000000000000, -1.000000000000000000 ) ) ;
#8565=ADVANCED_FACE ( 'NONE', ( #13524 ), #7502, .F. ) ;
#8566=CARTESIAN_POINT ( 'NONE',  ( 8.499999999999992895, 14.99364916731036956, 20.49999999999999645 ) ) ;
#8616=CARTESIAN_POINT ( 'NONE',  ( -13.00000000000000178, 15.00000000000000178, 25.00000000000000355 ) ) ;
#8620=EDGE_CURVE ( 'NONE', #17312, #2844, #7688, .T. ) ;
#8636=DIRECTION ( 'NONE',  ( -0.000000000000000000, 1.000000000000000000, -0.000000000000000000 ) ) ;
#8642=DIRECTION ( 'NONE',  ( -1.000000000000000000, 0.000000000000000000, 0.000000000000000000 ) ) ;
#8649=AXIS2_PLACEMENT_3D ( 'NONE', #11131, #9741, #15422 ) ;
#8651=CARTESIAN_POINT ( 'NONE',  ( -13.00000000000000178, 15.00000000000000178, -16.00000000000000000 ) ) ;
#8654=LINE ( 'NONE', #11261, #4062 ) ;
#8667=ORIENTED_EDGE ( 'NONE', *, *, #2688, .T. ) ;
#8673=DIRECTION ( 'NONE',  ( 0.000000000000000000, 0.000000000000000000, -1.000000000000000000 ) ) ;
#8681=EDGE_LOOP ( 'NONE', ( #9439, #10411 ) ) ;
#8742=EDGE_CURVE ( 'NONE', #12849, #16170, #17278, .T. ) ;
#8762=ORIENTED_EDGE ( 'NONE', *, *, #3041, .F. ) ;
#8807=AXIS2_PLACEMENT_3D ( 'NONE', #8329, #13904, #6935 ) ;
#8829=FACE_BOUND ( 'NONE', #9067, .T. ) ;
#8857=EDGE_CURVE ( 'NONE', #2215, #10311, #3790, .T. ) ;
#8903=VECTOR ( 'NONE', #452, 1000.000000000000000 ) ;
#8959=CIRCLE ( 'NONE', #10123, 2.200000000000000622 ) ;
#8962=CARTESIAN_POINT ( 'NONE',  ( 8.499999999999992895, 14.80000000000000071, 18.29999999999999716 ) ) ;
#8967=EDGE_CURVE ( 'NONE', #1285, #15329, #8165, .T. ) ;
#8969=AXIS2_PLACEMENT_3D ( 'NONE', #4831, #4918, #13166 ) ;
#8986=AXIS2_PLACEMENT_3D ( 'NONE', #10340, #3676, #2022 ) ;
#8999=EDGE_LOOP ( 'NONE', ( #11746, #800, #12211, #5173 ) ) ;
#9020=CARTESIAN_POINT ( 'NONE',  ( 12.00000000000000178, 48.00000000000000000, -15.00000000000000000 ) ) ;
#9024=CARTESIAN_POINT ( 'NONE',  ( 0.000000000000000000, 0.000000000000000000, 0.000000000000000000 ) ) ;
#9050=ORIENTED_EDGE ( 'NONE', *, *, #13460, .T. ) ;
#9065=CARTESIAN_POINT ( 'NONE',  ( 8.500000000000001776, 15.00000000000000000, -20.49999999999999645 ) ) ;
#9067=EDGE_LOOP ( 'NONE', ( #2481, #15038, #13597, #9733 ) ) ;
#9077=EDGE_CURVE ( 'NONE', #13832, #15656, #8492, .T. ) ;
#9141=APPLICATION_CONTEXT ( 'automotive_design' ) ;
#9146=ADVANCED_FACE ( 'NONE', ( #15932 ), #17711, .F. ) ;
#9147=CIRCLE ( 'NONE', #1166, 0.1999999999999987899 ) ;
#9260=VECTOR ( 'NONE', #12214, 1000.000000000000000 ) ;
#9270=ORIENTED_EDGE ( 'NONE', *, *, #10062, .F. ) ;
#9272=DIRECTION ( 'NONE',  ( 0.000000000000000000, 0.000000000000000000, -1.000000000000000000 ) ) ;
#9291=ORIENTED_EDGE ( 'NONE', *, *, #15618, .F. ) ;
#9347=VERTEX_POINT ( 'NONE', #8554 ) ;
#9372=AXIS2_PLACEMENT_3D ( 'NONE', #2577, #15277, #2669 ) ;
#9380=CARTESIAN_POINT ( 'NONE',  ( -8.500000000000005329, 13.00000000000000000, -18.35000000000000142 ) ) ;
#9439=ORIENTED_EDGE ( 'NONE', *, *, #8967, .F. ) ;
#9476=CIRCLE ( 'NONE', #5627, 2.149999999999995470 ) ;
#9481=CARTESIAN_POINT ( 'NONE',  ( 8.500000000000001776, 15.00000000000000178, -18.35000000000000142 ) ) ;
#9512=VERTEX_POINT ( 'NONE', #14827 ) ;
#9528=UNCERTAINTY_MEASURE_WITH_UNIT (LENGTH_MEASURE( 1.000000000000000082E-05 ), #1465, 'distance_accuracy_value', 'NONE');
#9532=DIRECTION ( 'NONE',  ( 0.000000000000000000, 0.000000000000000000, 1.000000000000000000 ) ) ;
#9538=PRODUCT_DEFINITION_FORMATION_WITH_SPECIFIED_SOURCE ( 'ANY', '', #6486, .NOT_KNOWN. ) ;
#9587=DIRECTION ( 'NONE',  ( -0.000000000000000000, 1.000000000000000000, -0.000000000000000000 ) ) ;
#9618=ORIENTED_EDGE ( 'NONE', *, *, #9800, .T. ) ;
#9657=ADVANCED_FACE ( 'NONE', ( #12564 ), #10840, .T. ) ;
#9663=AXIS2_PLACEMENT_3D ( 'NONE', #518, #4770, #10423 ) ;
#9670=CIRCLE ( 'NONE', #1696, 0.1999999999999987899 ) ;
#9684=LINE ( 'NONE', #8651, #3883 ) ;
#9686=LINE ( 'NONE', #4135, #13515 ) ;
#9688=DIRECTION ( 'NONE',  ( -1.000000000000000000, 0.000000000000000000, 0.000000000000000000 ) ) ;
#9695=AXIS2_PLACEMENT_3D ( 'NONE', #7549, #16104, #13203 ) ;
#9709=AXIS2_PLACEMENT_3D ( 'NONE', #17301, #3184, #11790 ) ;
#9723=AXIS2_PLACEMENT_3D ( 'NONE', #2420, #4823, #10471 ) ;
#9726=AXIS2_PLACEMENT_3D ( 'NONE', #10182, #15859, #4267 ) ;
#9727=EDGE_CURVE ( 'NONE', #17654, #6273, #6103, .T. ) ;
#9733=ORIENTED_EDGE ( 'NONE', *, *, #8620, .T. ) ;
#9741=DIRECTION ( 'NONE',  ( -1.000000000000000000, 0.000000000000000000, 0.000000000000000000 ) ) ;
#9757=FACE_OUTER_BOUND ( 'NONE', #7854, .T. ) ;
#9769=ADVANCED_FACE ( 'NONE', ( #6990 ), #16947, .F. ) ;
#9790=VERTEX_POINT ( 'NONE', #16766 ) ;
#9793=PRESENTATION_STYLE_ASSIGNMENT (( #4319 ) ) ;
#9800=EDGE_CURVE ( 'NONE', #9856, #6744, #9686, .T. ) ;
#9805=DIRECTION ( 'NONE',  ( -1.000000000000000000, 0.000000000000000000, -0.000000000000000000 ) ) ;
#9824=EDGE_CURVE ( 'NONE', #15656, #8139, #11259, .T. ) ;
#9825=( GEOMETRIC_REPRESENTATION_CONTEXT ( 3 ) GLOBAL_UNCERTAINTY_ASSIGNED_CONTEXT ( ( #9528 ) ) GLOBAL_UNIT_ASSIGNED_CONTEXT ( ( #1465, #13973, #12574 ) ) REPRESENTATION_CONTEXT ( 'NONE', 'WORKASPACE' ) );
#9837=DIRECTION ( 'NONE',  ( 0.000000000000000000, -1.000000000000000000, 0.000000000000000000 ) ) ;
#9856=VERTEX_POINT ( 'NONE', #10043 ) ;
#9863=ORIENTED_EDGE ( 'NONE', *, *, #7498, .T. ) ;
#9868=DIRECTION ( 'NONE',  ( 0.000000000000000000, 0.000000000000000000, -1.000000000000000000 ) ) ;
#9892=FACE_OUTER_BOUND ( 'NONE', #8999, .T. ) ;
#9900=DIRECTION ( 'NONE',  ( -0.000000000000000000, 1.000000000000000000, -0.000000000000000000 ) ) ;
#9910=CARTESIAN_POINT ( 'NONE',  ( 12.00000000000000178, 13.00000000000000178, -15.00000000000000000 ) ) ;
#9916=LINE ( 'NONE', #15423, #13565 ) ;
#9922=PLANE ( 'NONE',  #8052 ) ;
#9929=EDGE_CURVE ( 'NONE', #7280, #5293, #13020, .T. ) ;
#9931=CARTESIAN_POINT ( 'NONE',  ( 12.00000000000000178, 48.00000000000000000, 15.00000000000000000 ) ) ;
#9937=CARTESIAN_POINT ( 'NONE',  ( -13.00000000000000178, 13.00000000000000178, 25.00000000000000355 ) ) ;
#9941=FACE_OUTER_BOUND ( 'NONE', #3098, .T. ) ;
#9942=ORIENTED_EDGE ( 'NONE', *, *, #8857, .F. ) ;
#9965=PLANE ( 'NONE',  #6331 ) ;
#9981=ORIENTED_EDGE ( 'NONE', *, *, #13298, .T. ) ;
#9985=EDGE_LOOP ( 'NONE', ( #8230, #17134, #6097, #11274, #5487, #11548, #7353, #3770 ) ) ;
#9988=ADVANCED_FACE ( 'NONE', ( #4494 ), #16189, .T. ) ;
#10032=CIRCLE ( 'NONE', #12995, 2.149999999999995470 ) ;
#10033=LINE ( 'NONE', #41, #15749 ) ;
#10043=CARTESIAN_POINT ( 'NONE',  ( 13.00000000000000178, 15.00000000000000178, 25.00000000000000355 ) ) ;
#10046=LINE ( 'NONE', #1456, #13541 ) ;
#10056=CARTESIAN_POINT ( 'NONE',  ( -11.99999999999999822, 48.00000000000000000, 15.00000000000000000 ) ) ;
#10062=EDGE_CURVE ( 'NONE', #8139, #4992, #17602, .T. ) ;
#10107=DIRECTION ( 'NONE',  ( -0.000000000000000000, -1.000000000000000000, -0.000000000000000000 ) ) ;
#10123=AXIS2_PLACEMENT_3D ( 'NONE', #17430, #10534, #13223 ) ;
#10134=CARTESIAN_POINT ( 'NONE',  ( -13.00000000000000178, 15.00000000000000178, -25.00000000000000355 ) ) ;
#10182=CARTESIAN_POINT ( 'NONE',  ( 8.499999999999994671, 13.00000000000000000, 20.49999999999999645 ) ) ;
#10219=VECTOR ( 'NONE', #11321, 1000.000000000000000 ) ;
#10239=VERTEX_POINT ( 'NONE', #2909 ) ;
#10244=CARTESIAN_POINT ( 'NONE',  ( 13.00000000000000178, 48.00000000000000000, 16.00000000000000000 ) ) ;
#10264=CARTESIAN_POINT ( 'NONE',  ( -8.500000000000010658, 13.00000000000000000, 18.34999999999999432 ) ) ;
#10275=CARTESIAN_POINT ( 'NONE',  ( -11.99999999999999822, 13.00000000000000178, 15.00000000000000000 ) ) ;
#10306=EDGE_LOOP ( 'NONE', ( #3994, #1422, #13152, #15596 ) ) ;
#10311=VERTEX_POINT ( 'NONE', #9937 ) ;
#10340=CARTESIAN_POINT ( 'NONE',  ( 8.500000000000001776, 14.80000000000000071, -22.69999999999999929 ) ) ;
#10374=CARTESIAN_POINT ( 'NONE',  ( 8.499999999999992895, 14.99364916731036956, 20.49999999999999645 ) ) ;
#10383=DIRECTION ( 'NONE',  ( 1.000000000000000000, 0.000000000000000000, 0.000000000000000000 ) ) ;
#10404=DIRECTION ( 'NONE',  ( 0.000000000000000000, -0.000000000000000000, -1.000000000000000000 ) ) ;
#10410=DIRECTION ( 'NONE',  ( 0.000000000000000000, -0.000000000000000000, 1.000000000000000000 ) ) ;
#10411=ORIENTED_EDGE ( 'NONE', *, *, #3454, .F. ) ;
#10423=DIRECTION ( 'NONE',  ( 0.000000000000000000, 0.000000000000000000, 1.000000000000000000 ) ) ;
#10443=EDGE_LOOP ( 'NONE', ( #16379, #6422 ) ) ;
#10471=DIRECTION ( 'NONE',  ( 0.000000000000000000, 0.000000000000000000, 1.000000000000000000 ) ) ;
#10495=FACE_OUTER_BOUND ( 'NONE', #13400, .T. ) ;
#10519=AXIS2_PLACEMENT_3D ( 'NONE', #17098, #1602, #3084 ) ;
#10534=DIRECTION ( 'NONE',  ( -0.000000000000000000, 1.000000000000000000, -0.000000000000000000 ) ) ;
#10550=VECTOR ( 'NONE', #9868, 1000.000000000000000 ) ;
#10560=CARTESIAN_POINT ( 'NONE',  ( 0.000000000000000000, 48.00000000000000000, -16.00000000000000000 ) ) ;
#10561=EDGE_CURVE ( 'NONE', #297, #11364, #15908, .T. ) ;
#10589=LINE ( 'NONE', #14879, #1733 ) ;
#10592=ORIENTED_EDGE ( 'NONE', *, *, #16127, .T. ) ;
#10596=ORIENTED_EDGE ( 'NONE', *, *, #8742, .F. ) ;
#10603=AXIS2_PLACEMENT_3D ( 'NONE', #6963, #11228, #4280 ) ;
#10631=DIRECTION ( 'NONE',  ( 0.000000000000000000, 0.000000000000000000, 1.000000000000000000 ) ) ;
#10652=EDGE_CURVE ( 'NONE', #1285, #12849, #9670, .T. ) ;
#10677=CARTESIAN_POINT ( 'NONE',  ( -8.500000000000007105, 14.80000000000000071, -18.29999999999999716 ) ) ;
#10707=VERTEX_POINT ( 'NONE', #2535 ) ;
#10794=CARTESIAN_POINT ( 'NONE',  ( -8.500000000000010658, 13.00000000000000000, 20.49999999999998934 ) ) ;
#10806=EDGE_CURVE ( 'NONE', #11197, #10707, #15654, .T. ) ;
#10840=TOROIDAL_SURFACE ( 'NONE', #9372, 2.200000000000000178, 0.2000000000000000111 ) ;
#10877=SHAPE_REPRESENTATION ( 'Coil Housing', ( #16940 ), #16347 ) ;
#10926=ORIENTED_EDGE ( 'NONE', *, *, #11344, .F. ) ;
#10989=EDGE_LOOP ( 'NONE', ( #11048, #12089, #3042, #14264 ) ) ;
#11048=ORIENTED_EDGE ( 'NONE', *, *, #1677, .T. ) ;
#11073=LINE ( 'NONE', #18062, #13692 ) ;
#11080=DIRECTION ( 'NONE',  ( 0.000000000000000000, 0.000000000000000000, 1.000000000000000000 ) ) ;
#11107=ORIENTED_EDGE ( 'NONE', *, *, #6017, .T. ) ;
#11131=CARTESIAN_POINT ( 'NONE',  ( 12.00000000000000178, 48.00000000000000000, 15.00000000000000000 ) ) ;
#11148=LINE ( 'NONE', #13943, #13318 ) ;
#11158=CARTESIAN_POINT ( 'NONE',  ( -11.99999999999999822, 13.00000000000000178, -15.00000000000000000 ) ) ;
#11190=AXIS2_PLACEMENT_3D ( 'NONE', #11572, #5, #11669 ) ;
#11197=VERTEX_POINT ( 'NONE', #8122 ) ;
#11198=DIRECTION ( 'NONE',  ( 0.000000000000000000, -1.000000000000000000, 0.000000000000000000 ) ) ;
#11217=AXIS2_PLACEMENT_3D ( 'NONE', #16608, #1022, #9532 ) ;
#11227=FACE_OUTER_BOUND ( 'NONE', #12273, .T. ) ;
#11228=DIRECTION ( 'NONE',  ( -0.000000000000000000, 1.000000000000000000, -0.000000000000000000 ) ) ;
#11240=EDGE_CURVE ( 'NONE', #4895, #1346, #8654, .T. ) ;
#11248=ORIENTED_EDGE ( 'NONE', *, *, #13460, .F. ) ;
#11253=ORIENTED_EDGE ( 'NONE', *, *, #12494, .T. ) ;
#11259=LINE ( 'NONE', #4225, #10550 ) ;
#11261=CARTESIAN_POINT ( 'NONE',  ( 8.499999999999994671, 15.00000000000000178, 18.35000000000000142 ) ) ;
#11263=VERTEX_POINT ( 'NONE', #2671 ) ;
#11274=ORIENTED_EDGE ( 'NONE', *, *, #8295, .F. ) ;
#11298=CARTESIAN_POINT ( 'NONE',  ( 12.00000000000000178, 13.00000000000000178, 15.00000000000000000 ) ) ;
#11307=EDGE_CURVE ( 'NONE', #6836, #5293, #10046, .T. ) ;
#11309=ORIENTED_EDGE ( 'NONE', *, *, #8190, .F. ) ;
#11312=DIRECTION ( 'NONE',  ( 1.000000000000000000, 0.000000000000000000, 0.000000000000000000 ) ) ;
#11321=DIRECTION ( 'NONE',  ( -1.000000000000000000, -0.000000000000000000, -0.000000000000000000 ) ) ;
#11344=EDGE_CURVE ( 'NONE', #17654, #11263, #12649, .T. ) ;
#11345=CARTESIAN_POINT ( 'NONE',  ( 13.00000000000000178, 49.00000000000000000, -16.00000000000000000 ) ) ;
#11364=VERTEX_POINT ( 'NONE', #1361 ) ;
#11400=EDGE_LOOP ( 'NONE', ( #3334, #4891 ) ) ;
#11406=CARTESIAN_POINT ( 'NONE',  ( -13.00000000000000178, 13.00000000000000178, -25.00000000000000355 ) ) ;
#11422=DIRECTION ( 'NONE',  ( 0.000000000000000000, 0.000000000000000000, -1.000000000000000000 ) ) ;
#11430=DIRECTION ( 'NONE',  ( 0.000000000000000000, -1.000000000000000000, 0.000000000000000000 ) ) ;
#11446=DIRECTION ( 'NONE',  ( -0.000000000000000000, -1.000000000000000000, -0.000000000000000000 ) ) ;
#11457=CARTESIAN_POINT ( 'NONE',  ( -13.00000000000000178, 15.00000000000000178, -25.00000000000000355 ) ) ;
#11464=ADVANCED_FACE ( 'NONE', ( #15911 ), #17121, .T. ) ;
#11487=VECTOR ( 'NONE', #13831, 1000.000000000000000 ) ;
#11492=CARTESIAN_POINT ( 'NONE',  ( -8.500000000000010658, 14.99364916731036956, 20.49999999999998934 ) ) ;
#11538=ORIENTED_EDGE ( 'NONE', *, *, #842, .F. ) ;
#11548=ORIENTED_EDGE ( 'NONE', *, *, #4884, .T. ) ;
#11560=ORIENTED_EDGE ( 'NONE', *, *, #3601, .T. ) ;
#11572=CARTESIAN_POINT ( 'NONE',  ( 8.500000000000001776, 13.00000000000000000, -20.49999999999999645 ) ) ;
#11588=ORIENTED_EDGE ( 'NONE', *, *, #11344, .T. ) ;
#11603=AXIS2_PLACEMENT_3D ( 'NONE', #554, #14841, #6290 ) ;
#11609=CARTESIAN_POINT ( 'NONE',  ( 8.499999999999994671, 15.00000000000000178, 20.49999999999999645 ) ) ;
#11625=EDGE_CURVE ( 'NONE', #6401, #4895, #5260, .T. ) ;
#11652=AXIS2_PLACEMENT_3D ( 'NONE', #10560, #6113, #2058 ) ;
#11669=DIRECTION ( 'NONE',  ( 0.000000000000000000, 0.000000000000000000, 1.000000000000000000 ) ) ;
#11675=ORIENTED_EDGE ( 'NONE', *, *, #201, .T. ) ;
#11703=ADVANCED_FACE ( 'NONE', ( #17869 ), #16377, .F. ) ;
#11713=DIRECTION ( 'NONE',  ( -0.000000000000000000, -1.000000000000000000, -0.000000000000000000 ) ) ;
#11746=ORIENTED_EDGE ( 'NONE', *, *, #8620, .F. ) ;
#11750=ADVANCED_FACE ( 'NONE', ( #3933, #12087, #3665 ), #16463, .F. ) ;
#11790=DIRECTION ( 'NONE',  ( 0.000000000000000000, 0.000000000000000000, -1.000000000000000000 ) ) ;
#11796=DIRECTION ( 'NONE',  ( 0.000000000000000000, 1.000000000000000000, 0.000000000000000000 ) ) ;
#11809=EDGE_CURVE ( 'NONE', #3185, #5643, #13850, .T. ) ;
#11834=DIRECTION ( 'NONE',  ( -0.000000000000000000, 1.000000000000000000, -0.000000000000000000 ) ) ;
#11871=VECTOR ( 'NONE', #13307, 1000.000000000000000 ) ;
#11890=FACE_BOUND ( 'NONE', #8128, .T. ) ;
#11918=VECTOR ( 'NONE', #16316, 1000.000000000000000 ) ;
#11933=DIRECTION ( 'NONE',  ( -1.000000000000000000, 0.000000000000000000, -0.000000000000000000 ) ) ;
#11950=VECTOR ( 'NONE', #11446, 1000.000000000000000 ) ;
#11955=DIRECTION ( 'NONE',  ( 0.000000000000000000, 0.000000000000000000, -1.000000000000000000 ) ) ;
#11988=VECTOR ( 'NONE', #11713, 1000.000000000000000 ) ;
#11990=ADVANCED_FACE ( 'NONE', ( #15608 ), #1342, .F. ) ;
#12006=CARTESIAN_POINT ( 'NONE',  ( -13.00000000000000178, 49.00000000000000000, -16.00000000000000000 ) ) ;
#12019=CARTESIAN_POINT ( 'NONE',  ( 0.000000000000000000, 48.00000000000000000, 16.00000000000000000 ) ) ;
#12040=EDGE_CURVE ( 'NONE', #4710, #9347, #12819, .T. ) ;
#12067=ORIENTED_EDGE ( 'NONE', *, *, #7161, .T. ) ;
#12069=LINE ( 'NONE', #9020, #16589 ) ;
#12087=FACE_BOUND ( 'NONE', #10443, .T. ) ;
#12089=ORIENTED_EDGE ( 'NONE', *, *, #10561, .T. ) ;
#12091=CARTESIAN_POINT ( 'NONE',  ( -8.500000000000010658, 15.00000000000000000, 18.29999999999999005 ) ) ;
#12120=LINE ( 'NONE', #13237, #11918 ) ;
#12125=ORIENTED_EDGE ( 'NONE', *, *, #8168, .T. ) ;
#12155=EDGE_CURVE ( 'NONE', #16507, #6514, #12372, .T. ) ;
#12206=VECTOR ( 'NONE', #2500, 1000.000000000000000 ) ;
#12211=ORIENTED_EDGE ( 'NONE', *, *, #10806, .T. ) ;
#12214=DIRECTION ( 'NONE',  ( -0.000000000000000000, 1.000000000000000000, -0.000000000000000000 ) ) ;
#12229=ORIENTED_EDGE ( 'NONE', *, *, #4651, .T. ) ;
#12232=CIRCLE ( 'NONE', #8986, 0.1999999999999987899 ) ;
#12244=CARTESIAN_POINT ( 'NONE',  ( 13.00000000000000178, 48.00000000000000000, -16.00000000000000000 ) ) ;
#12261=PRODUCT_DEFINITION_SHAPE ( 'NONE', 'NONE',  #5599 ) ;
#12273=EDGE_LOOP ( 'NONE', ( #14865, #8762, #7808, #7474 ) ) ;
#12280=SHAPE_DEFINITION_REPRESENTATION ( #12261, #10877 ) ;
#12286=ORIENTED_EDGE ( 'NONE', *, *, #15618, .T. ) ;
#12322=LINE ( 'NONE', #15308, #5387 ) ;
#12360=DIRECTION ( 'NONE',  ( -1.000000000000000000, 0.000000000000000000, -0.000000000000000000 ) ) ;
#12361=DIRECTION ( 'NONE',  ( -1.000000000000000000, 0.000000000000000000, 0.000000000000000000 ) ) ;
#12372=CIRCLE ( 'NONE', #9709, 2.149999999999995470 ) ;
#12386=AXIS2_PLACEMENT_3D ( 'NONE', #2063, #17742, #3534 ) ;
#12494=EDGE_CURVE ( 'NONE', #14506, #12849, #10589, .T. ) ;
#12496=CARTESIAN_POINT ( 'NONE',  ( -8.500000000000005329, 13.00000000000000000, -22.64999999999999147 ) ) ;
#12497=AXIS2_PLACEMENT_3D ( 'NONE', #2250, #3625, #7875 ) ;
#12564=FACE_OUTER_BOUND ( 'NONE', #10989, .T. ) ;
#12574=( NAMED_UNIT ( * ) SI_UNIT ( $, .STERADIAN. ) SOLID_ANGLE_UNIT ( ) );
#12603=EDGE_CURVE ( 'NONE', #15334, #16170, #9916, .T. ) ;
#12605=ADVANCED_FACE ( 'NONE', ( #6868 ), #3911, .F. ) ;
#12648=AXIS2_PLACEMENT_3D ( 'NONE', #9065, #9587, #4807 ) ;
#12649=CIRCLE ( 'NONE', #7013, 0.1999999999999987899 ) ;
#12650=EDGE_CURVE ( 'NONE', #16492, #3217, #11, .T. ) ;
#12661=PRODUCT_DEFINITION_CONTEXT ( 'detailed design', #4758, 'design' ) ;
#12663=ORIENTED_EDGE ( 'NONE', *, *, #8190, .T. ) ;
#12673=AXIS2_PLACEMENT_3D ( 'NONE', #7990, #1054, #6608 ) ;
#12676=EDGE_CURVE ( 'NONE', #2215, #9856, #14103, .T. ) ;
#12712=DIRECTION ( 'NONE',  ( 0.000000000000000000, 0.000000000000000000, -1.000000000000000000 ) ) ;
#12731=CARTESIAN_POINT ( 'NONE',  ( -13.00000000000000178, 15.00000000000000178, 16.00000000000000000 ) ) ;
#12739=CARTESIAN_POINT ( 'NONE',  ( -8.500000000000007105, 14.99364916731036956, -20.49999999999999645 ) ) ;
#12743=EDGE_LOOP ( 'NONE', ( #15644, #3038, #6933, #13168 ) ) ;
#12809=CARTESIAN_POINT ( 'NONE',  ( -13.00000000000000178, 15.00000000000000178, 16.00000000000000000 ) ) ;
#12819=LINE ( 'NONE', #4022, #5562 ) ;
#12822=ORIENTED_EDGE ( 'NONE', *, *, #11240, .F. ) ;
#12847=LINE ( 'NONE', #10244, #11950 ) ;
#12849=VERTEX_POINT ( 'NONE', #4633 ) ;
#12855=DIRECTION ( 'NONE',  ( 1.000000000000000000, 0.000000000000000000, 1.224646799147353207E-16 ) ) ;
#12863=ORIENTED_EDGE ( 'NONE', *, *, #17964, .F. ) ;
#12873=EDGE_LOOP ( 'NONE', ( #14653, #13221, #9291, #11675 ) ) ;
#12905=CYLINDRICAL_SURFACE ( 'NONE', #3837, 2.149999999999995470 ) ;
#12943=ADVANCED_FACE ( 'NONE', ( #386, #7509, #6310 ), #16240, .F. ) ;
#12963=CIRCLE ( 'NONE', #17131, 2.149999999999995470 ) ;
#12995=AXIS2_PLACEMENT_3D ( 'NONE', #10374, #6479, #11955 ) ;
#13003=FACE_BOUND ( 'NONE', #13981, .T. ) ;
#13020=LINE ( 'NONE', #5971, #14714 ) ;
#13021=DIRECTION ( 'NONE',  ( 0.000000000000000000, -1.000000000000000000, 0.000000000000000000 ) ) ;
#13063=ORIENTED_EDGE ( 'NONE', *, *, #7156, .F. ) ;
#13084=DIRECTION ( 'NONE',  ( 0.000000000000000000, 0.000000000000000000, -1.000000000000000000 ) ) ;
#13095=EDGE_LOOP ( 'NONE', ( #4778, #15712, #8667, #3818 ) ) ;
#13116=DIRECTION ( 'NONE',  ( 0.000000000000000000, 0.000000000000000000, -1.000000000000000000 ) ) ;
#13123=ORIENTED_EDGE ( 'NONE', *, *, #16535, .F. ) ;
#13129=VERTEX_POINT ( 'NONE', #1212 ) ;
#13145=ORIENTED_EDGE ( 'NONE', *, *, #9727, .T. ) ;
#13146=EDGE_LOOP ( 'NONE', ( #4266, #17055, #9270, #14379 ) ) ;
#13152=ORIENTED_EDGE ( 'NONE', *, *, #3601, .F. ) ;
#13166=DIRECTION ( 'NONE',  ( 0.000000000000000000, 0.000000000000000000, 1.000000000000000000 ) ) ;
#13168=ORIENTED_EDGE ( 'NONE', *, *, #3440, .F. ) ;
#13203=DIRECTION ( 'NONE',  ( 0.000000000000000000, 0.000000000000000000, 1.000000000000000000 ) ) ;
#13221=ORIENTED_EDGE ( 'NONE', *, *, #12040, .F. ) ;
#13223=DIRECTION ( 'NONE',  ( 0.000000000000000000, 0.000000000000000000, 1.000000000000000000 ) ) ;
#13224=CARTESIAN_POINT ( 'NONE',  ( -8.500000000000010658, 15.00000000000000178, 20.49999999999998934 ) ) ;
#13237=CARTESIAN_POINT ( 'NONE',  ( -8.500000000000010658, 15.00000000000000178, 22.64999999999998437 ) ) ;
#13247=ORIENTED_EDGE ( 'NONE', *, *, #5020, .T. ) ;
#13278=ADVANCED_FACE ( 'NONE', ( #2425 ), #4065, .T. ) ;
#13298=EDGE_CURVE ( 'NONE', #6273, #17654, #15933, .T. ) ;
#13307=DIRECTION ( 'NONE',  ( -0.000000000000000000, -1.000000000000000000, -0.000000000000000000 ) ) ;
#13318=VECTOR ( 'NONE', #1254, 1000.000000000000000 ) ;
#13324=DIRECTION ( 'NONE',  ( 0.000000000000000000, 0.000000000000000000, 1.000000000000000000 ) ) ;
#13327=FACE_OUTER_BOUND ( 'NONE', #7393, .T. ) ;
#13356=PLANE ( 'NONE',  #3944 ) ;
#13370=DIRECTION ( 'NONE',  ( 0.000000000000000000, 0.000000000000000000, -1.000000000000000000 ) ) ;
#13374=EDGE_LOOP ( 'NONE', ( #11560, #9942, #4337, #12863, #7104, #3598, #14429, #3340 ) ) ;
#13394=CARTESIAN_POINT ( 'NONE',  ( 13.00000000000000178, 48.00000000000000000, 0.000000000000000000 ) ) ;
#13400=EDGE_LOOP ( 'NONE', ( #14370, #3170, #55, #6849 ) ) ;
#13433=EDGE_LOOP ( 'NONE', ( #6473, #3904, #5759, #6658 ) ) ;
#13460=EDGE_CURVE ( 'NONE', #15329, #16170, #15344, .T. ) ;
#13515=VECTOR ( 'NONE', #15461, 1000.000000000000000 ) ;
#13524=FACE_OUTER_BOUND ( 'NONE', #13146, .T. ) ;
#13541=VECTOR ( 'NONE', #14333, 1000.000000000000000 ) ;
#13557=DIRECTION ( 'NONE',  ( 0.000000000000000000, 0.000000000000000000, 1.000000000000000000 ) ) ;
#13565=VECTOR ( 'NONE', #2889, 1000.000000000000000 ) ;
#13577=ORIENTED_EDGE ( 'NONE', *, *, #13638, .F. ) ;
#13592=CYLINDRICAL_SURFACE ( 'NONE', #6488, 2.149999999999995470 ) ;
#13597=ORIENTED_EDGE ( 'NONE', *, *, #7156, .T. ) ;
#13615=EDGE_CURVE ( 'NONE', #9512, #11364, #14136, .T. ) ;
#13638=EDGE_CURVE ( 'NONE', #2662, #10239, #2310, .T. ) ;
#13655=DIRECTION ( 'NONE',  ( 0.000000000000000000, 0.000000000000000000, 1.000000000000000000 ) ) ;
#13666=CARTESIAN_POINT ( 'NONE',  ( -8.500000000000010658, 14.99364916731036956, 20.49999999999998934 ) ) ;
#13692=VECTOR ( 'NONE', #6634, 1000.000000000000000 ) ;
#13704=EDGE_LOOP ( 'NONE', ( #16479, #9050, #1534, #17871 ) ) ;
#13721=VERTEX_POINT ( 'NONE', #7577 ) ;
#13769=CYLINDRICAL_SURFACE ( 'NONE', #4845, 2.149999999999995470 ) ;
#13786=ORIENTED_EDGE ( 'NONE', *, *, #14211, .T. ) ;
#13825=AXIS2_PLACEMENT_3D ( 'NONE', #6418, #593, #13370 ) ;
#13831=DIRECTION ( 'NONE',  ( 1.000000000000000000, 0.000000000000000000, 0.000000000000000000 ) ) ;
#13832=VERTEX_POINT ( 'NONE', #4295 ) ;
#13850=CIRCLE ( 'NONE', #4365, 2.149999999999995470 ) ;
#13867=ORIENTED_EDGE ( 'NONE', *, *, #7437, .F. ) ;
#13889=EDGE_LOOP ( 'NONE', ( #12822, #16862, #12229, #872 ) ) ;
#13904=DIRECTION ( 'NONE',  ( -0.000000000000000000, 1.000000000000000000, -0.000000000000000000 ) ) ;
#13943=CARTESIAN_POINT ( 'NONE',  ( -13.00000000000000178, 13.00000000000000178, 25.00000000000000355 ) ) ;
#13962=DIRECTION ( 'NONE',  ( 0.000000000000000000, 0.000000000000000000, 1.000000000000000000 ) ) ;
#13970=ADVANCED_FACE ( 'NONE', ( #7343, #13003, #11890, #15893, #3190, #8829 ), #7535, .F. ) ;
#13972=CIRCLE ( 'NONE', #965, 0.1999999999999987899 ) ;
#13973=( NAMED_UNIT ( * ) PLANE_ANGLE_UNIT ( ) SI_UNIT ( $, .RADIAN. ) );
#13978=ORIENTED_EDGE ( 'NONE', *, *, #6010, .F. ) ;
#13981=EDGE_LOOP ( 'NONE', ( #17390, #14289 ) ) ;
#13994=CARTESIAN_POINT ( 'NONE',  ( -8.500000000000010658, 15.00000000000000000, 20.49999999999998934 ) ) ;
#14013=FACE_OUTER_BOUND ( 'NONE', #7956, .T. ) ;
#14062=ORIENTED_EDGE ( 'NONE', *, *, #14608, .F. ) ;
#14070=CARTESIAN_POINT ( 'NONE',  ( -8.500000000000007105, 15.00000000000000000, -20.49999999999999645 ) ) ;
#14087=AXIS2_PLACEMENT_3D ( 'NONE', #4975, #14828, #10631 ) ;
#14101=CARTESIAN_POINT ( 'NONE',  ( -11.99999999999999822, 13.00000000000000178, 15.00000000000000000 ) ) ;
#14103=LINE ( 'NONE', #15327, #11487 ) ;
#14136=CIRCLE ( 'NONE', #18311, 2.149999999999995470 ) ;
#14166=DIRECTION ( 'NONE',  ( 1.000000000000000000, 0.000000000000000000, 0.000000000000000000 ) ) ;
#14182=ADVANCED_FACE ( 'NONE', ( #16734 ), #18334, .T. ) ;
#14211=EDGE_CURVE ( 'NONE', #15334, #14506, #12963, .T. ) ;
#14261=DIRECTION ( 'NONE',  ( -1.000000000000000000, -0.000000000000000000, -0.000000000000000000 ) ) ;
#14264=ORIENTED_EDGE ( 'NONE', *, *, #2652, .F. ) ;
#14289=ORIENTED_EDGE ( 'NONE', *, *, #6934, .T. ) ;
#14324=ORIENTED_EDGE ( 'NONE', *, *, #16762, .T. ) ;
#14333=DIRECTION ( 'NONE',  ( -1.000000000000000000, 0.000000000000000000, -0.000000000000000000 ) ) ;
#14358=ORIENTED_EDGE ( 'NONE', *, *, #14897, .F. ) ;
#14359=ORIENTED_EDGE ( 'NONE', *, *, #16511, .F. ) ;
#14367=ORIENTED_EDGE ( 'NONE', *, *, #6992, .F. ) ;
#14370=ORIENTED_EDGE ( 'NONE', *, *, #9824, .T. ) ;
#14379=ORIENTED_EDGE ( 'NONE', *, *, #8295, .T. ) ;
#14418=LINE ( 'NONE', #12244, #11988 ) ;
#14424=CARTESIAN_POINT ( 'NONE',  ( -8.500000000000010658, 14.80000000000000071, 20.49999999999998934 ) ) ;
#14429=ORIENTED_EDGE ( 'NONE', *, *, #8168, .F. ) ;
#14473=ORIENTED_EDGE ( 'NONE', *, *, #2613, .F. ) ;
#14500=ADVANCED_FACE ( 'NONE', ( #15146 ), #4391, .T. ) ;
#14506=VERTEX_POINT ( 'NONE', #9380 ) ;
#14556=ORIENTED_EDGE ( 'NONE', *, *, #5910, .F. ) ;
#14599=ORIENTED_EDGE ( 'NONE', *, *, #6934, .F. ) ;
#14608=EDGE_CURVE ( 'NONE', #5643, #3185, #17760, .T. ) ;
#14653=ORIENTED_EDGE ( 'NONE', *, *, #6107, .T. ) ;
#14676=CARTESIAN_POINT ( 'NONE',  ( 13.00000000000000178, 15.00000000000000178, -25.00000000000000355 ) ) ;
#14714=VECTOR ( 'NONE', #1819, 1000.000000000000000 ) ;
#14744=VECTOR ( 'NONE', #6776, 1000.000000000000000 ) ;
#14827=CARTESIAN_POINT ( 'NONE',  ( -8.500000000000010658, 14.99364916731036956, 22.64999999999998437 ) ) ;
#14828=DIRECTION ( 'NONE',  ( -0.000000000000000000, 1.000000000000000000, -0.000000000000000000 ) ) ;
#14830=EDGE_CURVE ( 'NONE', #8268, #2949, #15836, .T. ) ;
#14838=AXIS2_PLACEMENT_3D ( 'NONE', #15394, #16879, #17912 ) ;
#14841=DIRECTION ( 'NONE',  ( -0.000000000000000000, 1.000000000000000000, -0.000000000000000000 ) ) ;
#14865=ORIENTED_EDGE ( 'NONE', *, *, #16477, .T. ) ;
#14879=CARTESIAN_POINT ( 'NONE',  ( -8.500000000000005329, 15.00000000000000178, -18.35000000000000142 ) ) ;
#14897=EDGE_CURVE ( 'NONE', #6273, #1346, #9147, .T. ) ;
#14916=CIRCLE ( 'NONE', #3635, 2.200000000000000622 ) ;
#14928=VECTOR ( 'NONE', #11312, 1000.000000000000000 ) ;
#14967=ADVANCED_FACE ( 'NONE', ( #1942 ), #13592, .F. ) ;
#14969=CARTESIAN_POINT ( 'NONE',  ( 0.000000000000000000, 49.00000000000000000, 0.000000000000000000 ) ) ;
#14986=CIRCLE ( 'NONE', #10519, 2.149999999999995470 ) ;
#14995=FACE_OUTER_BOUND ( 'NONE', #4385, .T. ) ;
#15038=ORIENTED_EDGE ( 'NONE', *, *, #11307, .T. ) ;
#15055=AXIS2_PLACEMENT_3D ( 'NONE', #14424, #7458, #3209 ) ;
#15068=DIRECTION ( 'NONE',  ( -0.000000000000000000, 0.000000000000000000, 1.000000000000000000 ) ) ;
#15098=ADVANCED_FACE ( 'NONE', ( #16487 ), #3765, .F. ) ;
#15115=CARTESIAN_POINT ( 'NONE',  ( -13.00000000000000178, 15.00000000000000178, 25.00000000000000355 ) ) ;
#15124=ORIENTED_EDGE ( 'NONE', *, *, #9077, .F. ) ;
#15146=FACE_OUTER_BOUND ( 'NONE', #13095, .T. ) ;
#15160=DIRECTION ( 'NONE',  ( -1.000000000000000000, -0.000000000000000000, -0.000000000000000000 ) ) ;
#15163=CARTESIAN_POINT ( 'NONE',  ( 8.500000000000001776, 14.99364916731036956, -18.35000000000000142 ) ) ;
#15277=DIRECTION ( 'NONE',  ( -0.000000000000000000, 1.000000000000000000, -0.000000000000000000 ) ) ;
#15308=CARTESIAN_POINT ( 'NONE',  ( 13.00000000000000178, 15.00000000000000178, 25.00000000000000355 ) ) ;
#15327=CARTESIAN_POINT ( 'NONE',  ( -13.00000000000000178, 15.00000000000000178, 25.00000000000000355 ) ) ;
#15329=VERTEX_POINT ( 'NONE', #18273 ) ;
#15334=VERTEX_POINT ( 'NONE', #12496 ) ;
#15344=CIRCLE ( 'NONE', #1720, 0.1999999999999987899 ) ;
#15345=AXIS2_PLACEMENT_3D ( 'NONE', #13394, #12361, #6530 ) ;
#15348=ADVANCED_FACE ( 'NONE', ( #9892 ), #7110, .T. ) ;
#15351=DIRECTION ( 'NONE',  ( -0.000000000000000000, 1.000000000000000000, -0.000000000000000000 ) ) ;
#15356=CIRCLE ( 'NONE', #16537, 2.149999999999995470 ) ;
#15394=CARTESIAN_POINT ( 'NONE',  ( -8.500000000000007105, 14.99364916731036956, -20.49999999999999645 ) ) ;
#15422=DIRECTION ( 'NONE',  ( 0.000000000000000000, 0.000000000000000000, 1.000000000000000000 ) ) ;
#15423=CARTESIAN_POINT ( 'NONE',  ( -8.500000000000005329, 15.00000000000000178, -22.64999999999999147 ) ) ;
#15454=ORIENTED_EDGE ( 'NONE', *, *, #12603, .F. ) ;
#15461=DIRECTION ( 'NONE',  ( -0.000000000000000000, -0.000000000000000000, -1.000000000000000000 ) ) ;
#15492=DIRECTION ( 'NONE',  ( -0.000000000000000000, -1.000000000000000000, -0.000000000000000000 ) ) ;
#15515=DIRECTION ( 'NONE',  ( -0.000000000000000000, 1.000000000000000000, -0.000000000000000000 ) ) ;
#15521=LINE ( 'NONE', #11406, #10219 ) ;
#15523=AXIS2_PLACEMENT_3D ( 'NONE', #8000, #6619, #13655 ) ;
#15532=ORIENTED_EDGE ( 'NONE', *, *, #2242, .T. ) ;
#15541=DIRECTION ( 'NONE',  ( -0.000000000000000000, -0.000000000000000000, 1.000000000000000000 ) ) ;
#15580=ORIENTED_EDGE ( 'NONE', *, *, #11307, .F. ) ;
#15594=CARTESIAN_POINT ( 'NONE',  ( -8.500000000000007105, 15.00000000000000000, -18.29999999999999716 ) ) ;
#15595=CARTESIAN_POINT ( 'NONE',  ( -8.500000000000005329, 13.00000000000000000, -20.49999999999999645 ) ) ;
#15596=ORIENTED_EDGE ( 'NONE', *, *, #6107, .F. ) ;
#15608=FACE_OUTER_BOUND ( 'NONE', #17041, .T. ) ;
#15618=EDGE_CURVE ( 'NONE', #2949, #4710, #4520, .T. ) ;
#15629=CARTESIAN_POINT ( 'NONE',  ( 8.499999999999994671, 15.00000000000000178, 20.49999999999999645 ) ) ;
#15632=CLOSED_SHELL ( 'NONE', ( #9657, #14182, #1113, #9988, #12605, #9146, #789, #15098, #11990, #9769, #5240, #14967, #8565, #15721, #13970, #11703, #2312, #2150, #6589, #4801, #15348, #13278, #16994, #1252, #11750, #8233, #12943, #5902, #14500, #1608, #11464 ) ) ;
#15644=ORIENTED_EDGE ( 'NONE', *, *, #11809, .F. ) ;
#15654=LINE ( 'NONE', #2954, #14744 ) ;
#15656=VERTEX_POINT ( 'NONE', #15839 ) ;
#15712=ORIENTED_EDGE ( 'NONE', *, *, #2383, .T. ) ;
#15721=ADVANCED_FACE ( 'NONE', ( #13327 ), #16398, .F. ) ;
#15749=VECTOR ( 'NONE', #15898, 1000.000000000000000 ) ;
#15836=LINE ( 'NONE', #17243, #1765 ) ;
#15839=CARTESIAN_POINT ( 'NONE',  ( 13.00000000000000178, 49.00000000000000000, 16.00000000000000000 ) ) ;
#15845=DIRECTION ( 'NONE',  ( 0.000000000000000000, 0.000000000000000000, -1.000000000000000000 ) ) ;
#15859=DIRECTION ( 'NONE',  ( -0.000000000000000000, 1.000000000000000000, -0.000000000000000000 ) ) ;
#15893=FACE_BOUND ( 'NONE', #11400, .T. ) ;
#15898=DIRECTION ( 'NONE',  ( 0.000000000000000000, 0.000000000000000000, 1.000000000000000000 ) ) ;
#15901=ORIENTED_EDGE ( 'NONE', *, *, #9929, .F. ) ;
#15908=CIRCLE ( 'NONE', #13825, 0.1999999999999987899 ) ;
#15911=FACE_OUTER_BOUND ( 'NONE', #13433, .T. ) ;
#15932=FACE_OUTER_BOUND ( 'NONE', #1884, .T. ) ;
#15933=CIRCLE ( 'NONE', #8807, 2.200000000000000622 ) ;
#16000=ORIENTED_EDGE ( 'NONE', *, *, #12603, .T. ) ;
#16029=DIRECTION ( 'NONE',  ( 0.000000000000000000, 0.000000000000000000, -1.000000000000000000 ) ) ;
#16055=DIRECTION ( 'NONE',  ( 1.000000000000000000, 0.000000000000000000, 0.000000000000000000 ) ) ;
#16058=MECHANICAL_DESIGN_GEOMETRIC_PRESENTATION_REPRESENTATION('',(#5679),#9825);
#16104=DIRECTION ( 'NONE',  ( -0.000000000000000000, 1.000000000000000000, -0.000000000000000000 ) ) ;
#16127=EDGE_CURVE ( 'NONE', #1346, #11263, #9476, .T. ) ;
#16135=EDGE_LOOP ( 'NONE', ( #12125, #15532, #1388, #12286 ) ) ;
#16163=CARTESIAN_POINT ( 'NONE',  ( 12.00000000000000178, 48.00000000000000000, 15.00000000000000000 ) ) ;
#16168=PLANE ( 'NONE',  #17200 ) ;
#16170=VERTEX_POINT ( 'NONE', #16186 ) ;
#16174=EDGE_LOOP ( 'NONE', ( #14358, #9981, #11588, #12067 ) ) ;
#16186=CARTESIAN_POINT ( 'NONE',  ( -8.500000000000005329, 14.99364916731036956, -22.64999999999999147 ) ) ;
#16189=TOROIDAL_SURFACE ( 'NONE', #9663, 2.200000000000000178, 0.2000000000000000111 ) ;
#16240=PLANE ( 'NONE',  #12386 ) ;
#16250=AXIS2_PLACEMENT_3D ( 'NONE', #2721, #8435, #18302 ) ;
#16278=VECTOR ( 'NONE', #658, 1000.000000000000000 ) ;
#16316=DIRECTION ( 'NONE',  ( -0.000000000000000000, 1.000000000000000000, -0.000000000000000000 ) ) ;
#16347=( GEOMETRIC_REPRESENTATION_CONTEXT ( 3 ) GLOBAL_UNCERTAINTY_ASSIGNED_CONTEXT ( ( #16605 ) ) GLOBAL_UNIT_ASSIGNED_CONTEXT ( ( #2229, #3778, #2408 ) ) REPRESENTATION_CONTEXT ( 'NONE', 'WORKASPACE' ) );
#16349=DIRECTION ( 'NONE',  ( -1.000000000000000000, 0.000000000000000000, 0.000000000000000000 ) ) ;
#16377=PLANE ( 'NONE',  #15345 ) ;
#16379=ORIENTED_EDGE ( 'NONE', *, *, #9727, .F. ) ;
#16398=PLANE ( 'NONE',  #7675 ) ;
#16408=ORIENTED_EDGE ( 'NONE', *, *, #12155, .F. ) ;
#16414=ORIENTED_EDGE ( 'NONE', *, *, #8742, .T. ) ;
#16450=DIRECTION ( 'NONE',  ( -0.000000000000000000, 1.000000000000000000, -0.000000000000000000 ) ) ;
#16463=PLANE ( 'NONE',  #18019 ) ;
#16477=EDGE_CURVE ( 'NONE', #10311, #16492, #11148, .T. ) ;
#16479=ORIENTED_EDGE ( 'NONE', *, *, #8967, .T. ) ;
#16486=AXIS2_PLACEMENT_3D ( 'NONE', #8386, #6820, #1183 ) ;
#16487=FACE_OUTER_BOUND ( 'NONE', #12743, .T. ) ;
#16492=VERTEX_POINT ( 'NONE', #16562 ) ;
#16507=VERTEX_POINT ( 'NONE', #15163 ) ;
#16511=EDGE_CURVE ( 'NONE', #9790, #7280, #1341, .T. ) ;
#16535=EDGE_CURVE ( 'NONE', #3185, #11364, #2738, .T. ) ;
#16537=AXIS2_PLACEMENT_3D ( 'NONE', #12739, #3193, #11422 ) ;
#16547=CARTESIAN_POINT ( 'NONE',  ( 8.500000000000001776, 14.80000000000000071, -20.49999999999999645 ) ) ;
#16562=CARTESIAN_POINT ( 'NONE',  ( 13.00000000000000178, 13.00000000000000178, 25.00000000000000355 ) ) ;
#16589=VECTOR ( 'NONE', #1904, 1000.000000000000000 ) ;
#16605=UNCERTAINTY_MEASURE_WITH_UNIT (LENGTH_MEASURE( 1.000000000000000082E-05 ), #2229, 'distance_accuracy_value', 'NONE');
#16608=CARTESIAN_POINT ( 'NONE',  ( 8.500000000000001776, 13.00000000000000000, -20.49999999999999645 ) ) ;
#16656=CARTESIAN_POINT ( 'NONE',  ( -11.99999999999999822, 48.00000000000000000, -15.00000000000000000 ) ) ;
#16660=DIRECTION ( 'NONE',  ( 0.000000000000000000, 0.000000000000000000, -1.000000000000000000 ) ) ;
#16686=CARTESIAN_POINT ( 'NONE',  ( 8.499999999999994671, 15.00000000000000178, 22.64999999999999147 ) ) ;
#16698=ADVANCED_BREP_SHAPE_REPRESENTATION ( '', ( #2427, #16940 ), #16347 ) ;
#16734=FACE_OUTER_BOUND ( 'NONE', #17302, .T. ) ;
#16743=AXIS2_PLACEMENT_3D ( 'NONE', #10134, #7728, #3296 ) ;
#16754=LINE ( 'NONE', #1078, #4372 ) ;
#16762=EDGE_CURVE ( 'NONE', #3421, #2215, #4565, .T. ) ;
#16766=CARTESIAN_POINT ( 'NONE',  ( 12.00000000000000178, 48.00000000000000000, -15.00000000000000000 ) ) ;
#16821=CARTESIAN_POINT ( 'NONE',  ( 8.499999999999992895, 15.00000000000000000, 18.29999999999999716 ) ) ;
#16862=ORIENTED_EDGE ( 'NONE', *, *, #11625, .F. ) ;
#16863=CARTESIAN_POINT ( 'NONE',  ( 8.499999999999992895, 15.00000000000000000, 22.69999999999999929 ) ) ;
#16879=DIRECTION ( 'NONE',  ( 0.000000000000000000, -1.000000000000000000, 0.000000000000000000 ) ) ;
#16900=EDGE_LOOP ( 'NONE', ( #7215, #13786 ) ) ;
#16940=AXIS2_PLACEMENT_3D ( 'NONE', #9024, #13557, #6428 ) ;
#16947=CYLINDRICAL_SURFACE ( 'NONE', #1988, 2.149999999999995470 ) ;
#16950=DIRECTION ( 'NONE',  ( -0.000000000000000000, 1.000000000000000000, -0.000000000000000000 ) ) ;
#16994=ADVANCED_FACE ( 'NONE', ( #10495 ), #16168, .F. ) ;
#17029=CARTESIAN_POINT ( 'NONE',  ( 8.500000000000001776, 14.80000000000000071, -18.29999999999999716 ) ) ;
#17041=EDGE_LOOP ( 'NONE', ( #13123, #14062, #4755, #4817 ) ) ;
#17055=ORIENTED_EDGE ( 'NONE', *, *, #4237, .F. ) ;
#17090=DIRECTION ( 'NONE',  ( -1.000000000000000000, 0.000000000000000000, -0.000000000000000000 ) ) ;
#17098=CARTESIAN_POINT ( 'NONE',  ( -8.500000000000005329, 13.00000000000000000, -20.49999999999999645 ) ) ;
#17105=DIRECTION ( 'NONE',  ( 0.000000000000000000, 0.000000000000000000, 1.000000000000000000 ) ) ;
#17121=TOROIDAL_SURFACE ( 'NONE', #15055, 2.200000000000000178, 0.2000000000000000111 ) ;
#17131=AXIS2_PLACEMENT_3D ( 'NONE', #15595, #15515, #2812 ) ;
#17134=ORIENTED_EDGE ( 'NONE', *, *, #201, .F. ) ;
#17177=VECTOR ( 'NONE', #14261, 1000.000000000000000 ) ;
#17193=VECTOR ( 'NONE', #6972, 1000.000000000000000 ) ;
#17196=CARTESIAN_POINT ( 'NONE',  ( 13.00000000000000178, 15.00000000000000000, 16.00000000000000000 ) ) ;
#17200=AXIS2_PLACEMENT_3D ( 'NONE', #14969, #2266, #10404 ) ;
#17239=AXIS2_PLACEMENT_3D ( 'NONE', #16547, #16450, #4010 ) ;
#17243=CARTESIAN_POINT ( 'NONE',  ( 13.00000000000000178, 15.00000000000000178, -16.00000000000000000 ) ) ;
#17250=AXIS2_PLACEMENT_3D ( 'NONE', #17308, #221, #1618 ) ;
#17278=CIRCLE ( 'NONE', #14838, 2.149999999999995470 ) ;
#17293=EDGE_CURVE ( 'NONE', #4992, #13832, #5756, .T. ) ;
#17301=CARTESIAN_POINT ( 'NONE',  ( 8.500000000000001776, 14.99364916731036956, -20.49999999999999645 ) ) ;
#17302=EDGE_LOOP ( 'NONE', ( #13145, #1914, #10592, #10926 ) ) ;
#17308=CARTESIAN_POINT ( 'NONE',  ( -8.500000000000010658, 14.80000000000000071, 22.69999999999999218 ) ) ;
#17312=VERTEX_POINT ( 'NONE', #14101 ) ;
#17348=CARTESIAN_POINT ( 'NONE',  ( -13.00000000000000178, 49.00000000000000000, 16.00000000000000000 ) ) ;
#17366=VECTOR ( 'NONE', #13084, 1000.000000000000000 ) ;
#17372=CARTESIAN_POINT ( 'NONE',  ( -12.99999999999999822, 48.00000000000000000, 0.000000000000000000 ) ) ;
#17387=DIRECTION ( 'NONE',  ( 0.000000000000000000, 0.000000000000000000, 1.000000000000000000 ) ) ;
#17390=ORIENTED_EDGE ( 'NONE', *, *, #7437, .T. ) ;
#17391=ORIENTED_EDGE ( 'NONE', *, *, #1677, .F. ) ;
#17430=CARTESIAN_POINT ( 'NONE',  ( -8.500000000000010658, 15.00000000000000000, 20.49999999999998934 ) ) ;
#17441=PLANE ( 'NONE',  #8649 ) ;
#17446=CARTESIAN_POINT ( 'NONE',  ( 8.500000000000001776, 13.00000000000000000, -18.34999999999999787 ) ) ;
#17464=ORIENTED_EDGE ( 'NONE', *, *, #7037, .F. ) ;
#17602=LINE ( 'NONE', #3838, #4035 ) ;
#17636=ORIENTED_EDGE ( 'NONE', *, *, #3454, .T. ) ;
#17650=CARTESIAN_POINT ( 'NONE',  ( -11.99999999999999822, 13.00000000000000178, 15.00000000000000000 ) ) ;
#17654=VERTEX_POINT ( 'NONE', #16863 ) ;
#17700=PRODUCT_CONTEXT ( 'NONE', #9141, 'mechanical' ) ;
#17711=CYLINDRICAL_SURFACE ( 'NONE', #14087, 2.149999999999995470 ) ;
#17721=EDGE_LOOP ( 'NONE', ( #15454, #13978, #11253, #5551 ) ) ;
#17742=DIRECTION ( 'NONE',  ( 0.000000000000000000, -1.000000000000000000, 0.000000000000000000 ) ) ;
#17760=CIRCLE ( 'NONE', #9723, 2.149999999999995470 ) ;
#17771=EDGE_LOOP ( 'NONE', ( #11248, #17636, #1468, #16414 ) ) ;
#17783=AXIS2_PLACEMENT_3D ( 'NONE', #5371, #6752, #9805 ) ;
#17864=AXIS2_PLACEMENT_3D ( 'NONE', #1271, #11430, #8562 ) ;
#17869=FACE_OUTER_BOUND ( 'NONE', #9985, .T. ) ;
#17871=ORIENTED_EDGE ( 'NONE', *, *, #10652, .F. ) ;
#17878=CIRCLE ( 'NONE', #8969, 2.200000000000000622 ) ;
#17879=CARTESIAN_POINT ( 'NONE',  ( 8.500000000000001776, 15.00000000000000178, -20.49999999999999645 ) ) ;
#17886=DIRECTION ( 'NONE',  ( -0.000000000000000000, 1.000000000000000000, -0.000000000000000000 ) ) ;
#17895=ORIENTED_EDGE ( 'NONE', *, *, #11625, .T. ) ;
#17912=DIRECTION ( 'NONE',  ( 0.000000000000000000, 0.000000000000000000, -1.000000000000000000 ) ) ;
#17938=ORIENTED_EDGE ( 'NONE', *, *, #4651, .F. ) ;
#17964=EDGE_CURVE ( 'NONE', #13832, #3421, #7917, .T. ) ;
#18019=AXIS2_PLACEMENT_3D ( 'NONE', #2378, #6708, #706 ) ;
#18062=CARTESIAN_POINT ( 'NONE',  ( 8.500000000000001776, 15.00000000000000178, -22.64999999999999147 ) ) ;
#18161=CIRCLE ( 'NONE', #6575, 2.149999999999995470 ) ;
#18175=CARTESIAN_POINT ( 'NONE',  ( -12.99999999999999822, 13.00000000000000178, 0.000000000000000000 ) ) ;
#18263=UNCERTAINTY_MEASURE_WITH_UNIT (LENGTH_MEASURE( 1.000000000000000082E-05 ), #2338, 'distance_accuracy_value', 'NONE');
#18269=VECTOR ( 'NONE', #2421, 1000.000000000000000 ) ;
#18273=CARTESIAN_POINT ( 'NONE',  ( -8.500000000000007105, 15.00000000000000000, -22.69999999999999929 ) ) ;
#18302=DIRECTION ( 'NONE',  ( 0.000000000000000000, 0.000000000000000000, 1.000000000000000000 ) ) ;
#18311=AXIS2_PLACEMENT_3D ( 'NONE', #13666, #2563, #16660 ) ;
#18334=TOROIDAL_SURFACE ( 'NONE', #10603, 2.200000000000000178, 0.2000000000000000111 ) ;
#18383=COLOUR_RGB('Dark Blue',0.08,0.2,0.34);
#18384=FILL_AREA_STYLE_COLOUR('',#18383);
#18385=FILL_AREA_STYLE('',(#18384));
#18386=SURFACE_STYLE_FILL_AREA(#18385);
#18387=SURFACE_SIDE_STYLE('',(#18386));
#18388=SURFACE_STYLE_USAGE(.BOTH.,#18387);
#18389=PRESENTATION_STYLE_ASSIGNMENT((#18388));
ENDSEC;
END-ISO-10303-21;
